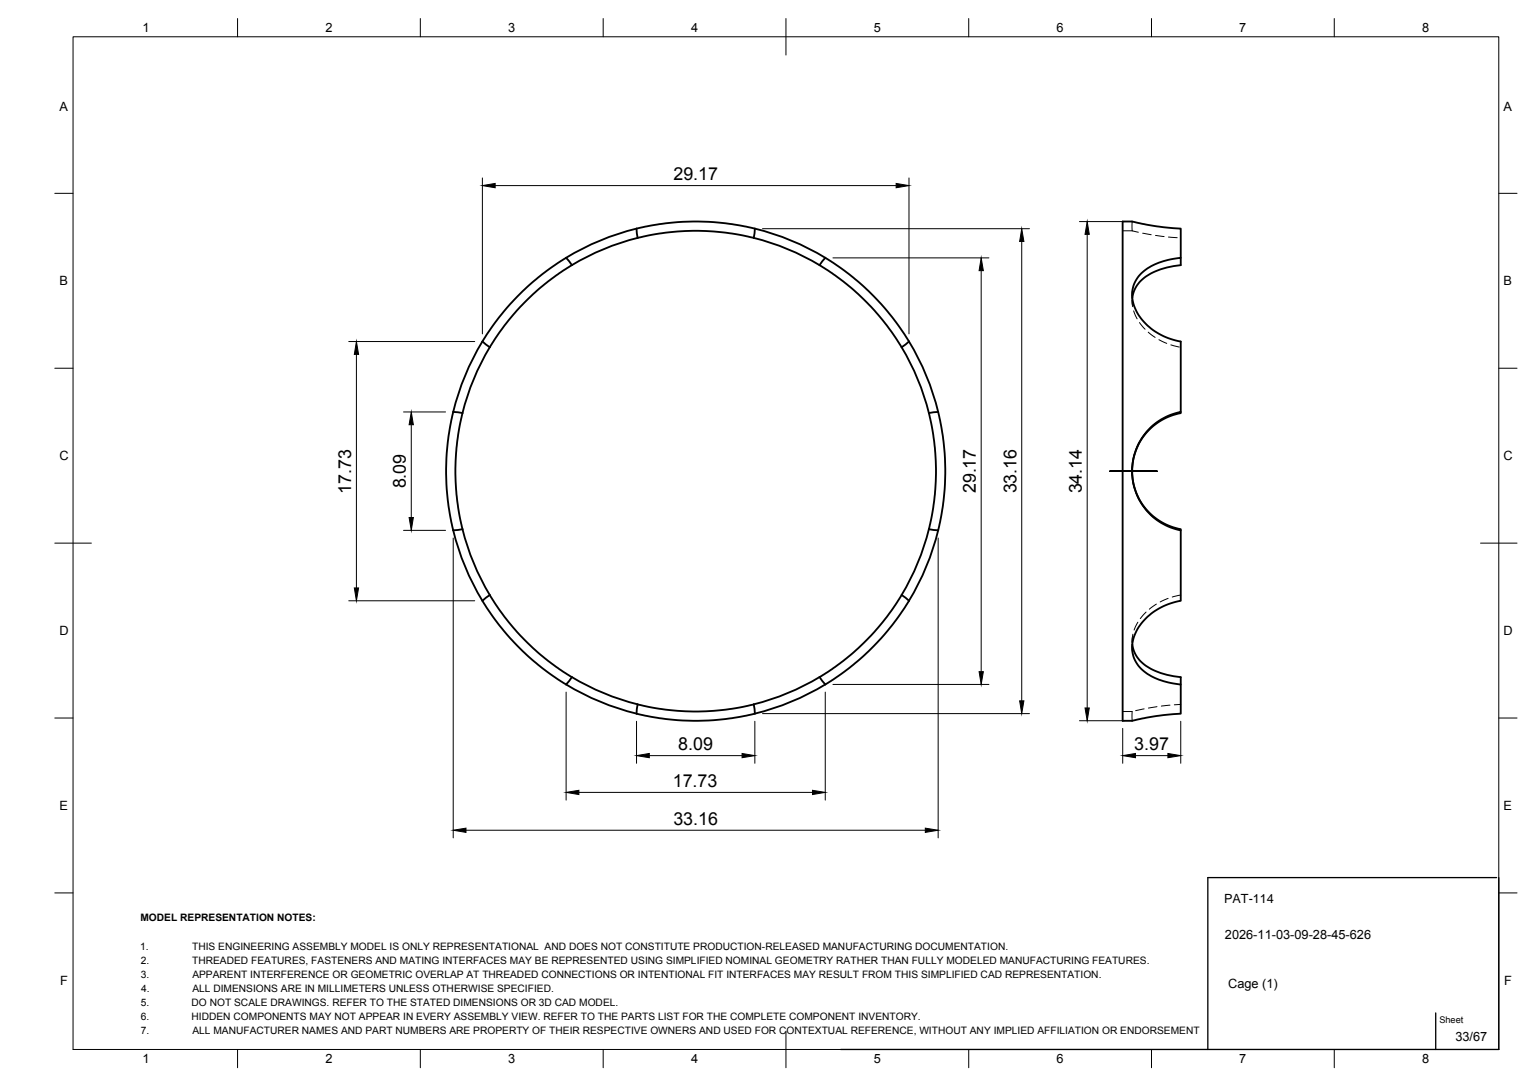
ISO-10303-21;
HEADER;
/* Generated by software containing ST-Developer
 * from STEP Tools, Inc. (www.steptools.com) 
 */

FILE_DESCRIPTION(
/* description */ ('Two-stage gear reducer in split housing'),
/* implementation_level */ '2;1');

FILE_NAME(
/* name */ 'Cage (1).step',
/* time_stamp */ '2026-10-28T03:22:31-07:00',
/* author */ (''),
/* organization */ (''),
/* preprocessor_version */ 'ST-DEVELOPER v20.2',
/* originating_system */ 'Autodesk Translation Framework v15.17.0.0',
/* authorisation */ '');

FILE_SCHEMA (('AUTOMOTIVE_DESIGN { 1 0 10303 214 3 1 1 }'));
ENDSEC;

DATA;
#10=MECHANICAL_DESIGN_GEOMETRIC_PRESENTATION_REPRESENTATION('',(#1273),#73366);
#945=B_SPLINE_CURVE_WITH_KNOTS('',3,(#24814,#24815,#24816,#24817,#24818,
#24819,#24820,#24821,#24822,#24823,#24824,#24825,#24826,#24827,#24828,#24829,
#24830,#24831,#24832,#24833,#24834,#24835),.UNSPECIFIED.,.F.,.F.,(4,2,2,
2,2,2,2,2,2,2,4),(0.0789094028588958,0.210573405340968,0.315860108011452,
0.421146810681936,0.522142632548711,0.623138454415485,0.72413427628226,
0.825130098149035,0.930416800819519,1.03570350349,1.16736750597208),
 .UNSPECIFIED.);
#946=B_SPLINE_CURVE_WITH_KNOTS('',3,(#24839,#24840,#24841,#24842,#24843,
#24844,#24845,#24846,#24847,#24848,#24849,#24850,#24851,#24852,#24853,#24854,
#24855,#24856,#24857,#24858,#24859,#24860),.UNSPECIFIED.,.F.,.F.,(4,2,2,
2,2,2,2,2,2,2,4),(0.0774793363974613,0.142088896491891,0.284177792983782,
0.411119756996526,0.514392970548519,0.617666184100513,0.720939397652506,
0.8242126112045,0.951154575217244,1.09324347170913,1.15785303180356),
 .UNSPECIFIED.);
#947=B_SPLINE_CURVE_WITH_KNOTS('',3,(#24866,#24867,#24868,#24869,#24870,
#24871,#24872,#24873,#24874,#24875,#24876,#24877,#24878,#24879,#24880,#24881,
#24882,#24883,#24884,#24885,#24886,#24887),.UNSPECIFIED.,.F.,.F.,(4,2,2,
2,2,2,2,2,2,2,4),(0.0774793363974613,0.142088896491891,0.284177792983782,
0.411119756996525,0.514392970548519,0.617666184100513,0.720939397652506,
0.8242126112045,0.951154575217243,1.09324347170913,1.15785303180356),
 .UNSPECIFIED.);
#948=B_SPLINE_CURVE_WITH_KNOTS('',3,(#24891,#24892,#24893,#24894,#24895,
#24896,#24897,#24898,#24899,#24900,#24901,#24902,#24903,#24904,#24905,#24906,
#24907,#24908,#24909,#24910,#24911,#24912),.UNSPECIFIED.,.F.,.F.,(4,2,2,
2,2,2,2,2,2,2,4),(0.0774793363974614,0.142088896491891,0.284177792983781,
0.411119756996525,0.514392970548519,0.617666184100512,0.720939397652506,
0.824212611204499,0.951154575217243,1.09324347170913,1.15785303180356),
 .UNSPECIFIED.);
#949=B_SPLINE_CURVE_WITH_KNOTS('',3,(#24916,#24917,#24918,#24919,#24920,
#24921,#24922,#24923,#24924,#24925,#24926,#24927),.UNSPECIFIED.,.F.,.F.,
(4,2,2,2,2,4),(0.0774793363974613,0.142088896491891,0.284177792983781,0.411119756996525,
0.514392970548519,0.617666184100512),.UNSPECIFIED.);
#950=B_SPLINE_CURVE_WITH_KNOTS('',3,(#24932,#24933,#24934,#24935,#24936,
#24937,#24938,#24939,#24940,#24941,#24942,#24943),.UNSPECIFIED.,.F.,.F.,
(4,2,2,2,2,4),(0.617666184100512,0.720939397652506,0.824212611204499,0.951154575217243,
1.09324347170913,1.15785303180356),.UNSPECIFIED.);
#951=B_SPLINE_CURVE_WITH_KNOTS('',3,(#24947,#24948,#24949,#24950,#24951,
#24952,#24953,#24954,#24955,#24956,#24957,#24958,#24959,#24960,#24961,#24962,
#24963,#24964,#24965,#24966,#24967,#24968),.UNSPECIFIED.,.F.,.F.,(4,2,2,
2,2,2,2,2,2,2,4),(0.0774793363974613,0.142088896491891,0.284177792983782,
0.411119756996526,0.514392970548519,0.617666184100513,0.720939397652507,
0.8242126112045,0.951154575217245,1.09324347170914,1.15785303180356),
 .UNSPECIFIED.);
#952=B_SPLINE_CURVE_WITH_KNOTS('',3,(#24972,#24973,#24974,#24975,#24976,
#24977,#24978,#24979,#24980,#24981,#24982,#24983,#24984,#24985,#24986,#24987,
#24988,#24989,#24990,#24991,#24992,#24993),.UNSPECIFIED.,.F.,.F.,(4,2,2,
2,2,2,2,2,2,2,4),(0.0774793363974613,0.142088896491891,0.284177792983782,
0.411119756996526,0.514392970548519,0.617666184100513,0.720939397652506,
0.824212611204499,0.951154575217243,1.09324347170913,1.15785303180356),
 .UNSPECIFIED.);
#953=B_SPLINE_CURVE_WITH_KNOTS('',3,(#24997,#24998,#24999,#25000,#25001,
#25002,#25003,#25004,#25005,#25006,#25007,#25008,#25009,#25010,#25011,#25012,
#25013,#25014,#25015,#25016,#25017,#25018),.UNSPECIFIED.,.F.,.F.,(4,2,2,
2,2,2,2,2,2,2,4),(0.0774793363974613,0.142088896491891,0.284177792983782,
0.411119756996526,0.514392970548519,0.617666184100513,0.720939397652506,
0.8242126112045,0.951154575217244,1.09324347170913,1.15785303180356),
 .UNSPECIFIED.);
#954=B_SPLINE_CURVE_WITH_KNOTS('',3,(#25022,#25023,#25024,#25025,#25026,
#25027,#25028,#25029,#25030,#25031,#25032,#25033,#25034,#25035,#25036,#25037,
#25038,#25039,#25040,#25041,#25042,#25043),.UNSPECIFIED.,.F.,.F.,(4,2,2,
2,2,2,2,2,2,2,4),(0.0774793363974613,0.142088896491891,0.284177792983782,
0.411119756996526,0.514392970548519,0.617666184100513,0.720939397652506,
0.8242126112045,0.951154575217243,1.09324347170913,1.15785303180356),
 .UNSPECIFIED.);
#955=B_SPLINE_CURVE_WITH_KNOTS('',3,(#25051,#25052,#25053,#25054,#25055,
#25056,#25057,#25058,#25059,#25060,#25061,#25062,#25063,#25064,#25065,#25066,
#25067,#25068,#25069,#25070,#25071,#25072),.UNSPECIFIED.,.F.,.F.,(4,2,2,
2,2,2,2,2,2,2,4),(0.0789094028588958,0.210573405340968,0.315860108011452,
0.421146810681936,0.522142632548711,0.623138454415485,0.72413427628226,
0.825130098149035,0.930416800819519,1.03570350349,1.16736750597208),
 .UNSPECIFIED.);
#956=B_SPLINE_CURVE_WITH_KNOTS('',3,(#25080,#25081,#25082,#25083,#25084,
#25085,#25086,#25087,#25088,#25089,#25090,#25091,#25092,#25093,#25094,#25095,
#25096,#25097,#25098,#25099,#25100,#25101),.UNSPECIFIED.,.F.,.F.,(4,2,2,
2,2,2,2,2,2,2,4),(0.0789094028588958,0.210573405340969,0.315860108011453,
0.421146810681937,0.522142632548712,0.623138454415486,0.724134276282261,
0.825130098149035,0.930416800819519,1.03570350349,1.16736750597208),
 .UNSPECIFIED.);
#957=B_SPLINE_CURVE_WITH_KNOTS('',3,(#25110,#25111,#25112,#25113,#25114,
#25115,#25116,#25117,#25118,#25119,#25120,#25121),.UNSPECIFIED.,.F.,.F.,
(4,2,2,2,2,4),(0.0789094028588958,0.210573405340968,0.315860108011452,0.421146810681937,
0.522142632548711,0.623138454415486),.UNSPECIFIED.);
#958=B_SPLINE_CURVE_WITH_KNOTS('',3,(#25123,#25124,#25125,#25126,#25127,
#25128,#25129,#25130,#25131,#25132,#25133,#25134),.UNSPECIFIED.,.F.,.F.,
(4,2,2,2,2,4),(0.623138454415486,0.72413427628226,0.825130098149035,0.930416800819519,
1.03570350349,1.16736750597208),.UNSPECIFIED.);
#959=B_SPLINE_CURVE_WITH_KNOTS('',3,(#25141,#25142,#25143,#25144,#25145,
#25146,#25147,#25148,#25149,#25150,#25151,#25152,#25153,#25154,#25155,#25156,
#25157,#25158,#25159,#25160,#25161,#25162),.UNSPECIFIED.,.F.,.F.,(4,2,2,
2,2,2,2,2,2,2,4),(0.0789094028588958,0.210573405340968,0.315860108011452,
0.421146810681936,0.522142632548711,0.623138454415486,0.72413427628226,
0.825130098149035,0.930416800819519,1.03570350349,1.16736750597208),
 .UNSPECIFIED.);
#960=B_SPLINE_CURVE_WITH_KNOTS('',3,(#25170,#25171,#25172,#25173,#25174,
#25175,#25176,#25177,#25178,#25179,#25180,#25181,#25182,#25183,#25184,#25185,
#25186,#25187,#25188,#25189,#25190,#25191),.UNSPECIFIED.,.F.,.F.,(4,2,2,
2,2,2,2,2,2,2,4),(0.0789094028588957,0.210573405340968,0.315860108011452,
0.421146810681936,0.522142632548711,0.623138454415485,0.72413427628226,
0.825130098149035,0.930416800819519,1.03570350349,1.16736750597207),
 .UNSPECIFIED.);
#961=B_SPLINE_CURVE_WITH_KNOTS('',3,(#25199,#25200,#25201,#25202,#25203,
#25204,#25205,#25206,#25207,#25208,#25209,#25210,#25211,#25212,#25213,#25214,
#25215,#25216,#25217,#25218,#25219,#25220),.UNSPECIFIED.,.F.,.F.,(4,2,2,
2,2,2,2,2,2,2,4),(0.0789094028588958,0.210573405340968,0.315860108011452,
0.421146810681936,0.522142632548711,0.623138454415486,0.72413427628226,
0.825130098149035,0.930416800819519,1.03570350349,1.16736750597208),
 .UNSPECIFIED.);
#962=B_SPLINE_CURVE_WITH_KNOTS('',3,(#25229,#25230,#25231,#25232,#25233,
#25234,#25235,#25236,#25237,#25238,#25239,#25240,#25241,#25242,#25243,#25244,
#25245,#25246,#25247,#25248,#25249,#25250),.UNSPECIFIED.,.F.,.F.,(4,2,2,
2,2,2,2,2,2,2,4),(0.0789094028588958,0.210573405340968,0.315860108011452,
0.421146810681936,0.522142632548711,0.623138454415485,0.72413427628226,
0.825130098149035,0.930416800819519,1.03570350349,1.16736750597208),
 .UNSPECIFIED.);
#1089=SPHERICAL_SURFACE('',#17603,0.412776);
#1090=SPHERICAL_SURFACE('',#17619,0.412776);
#1091=SPHERICAL_SURFACE('',#17624,0.412776);
#1092=SPHERICAL_SURFACE('',#17629,0.412776);
#1093=SPHERICAL_SURFACE('',#17634,0.412776);
#1094=SPHERICAL_SURFACE('',#17639,0.412776);
#1095=SPHERICAL_SURFACE('',#17644,0.412776);
#1096=SPHERICAL_SURFACE('',#17652,0.412776);
#1147=SHAPE_REPRESENTATION_RELATIONSHIP('SRR','None',#73636,#1203);
#1203=ADVANCED_BREP_SHAPE_REPRESENTATION('',(#1343),#73332);
#1273=STYLED_ITEM('',(#73988),#1343);
#1343=MANIFOLD_SOLID_BREP('Continuous crown cage',#16162);
#1532=FACE_BOUND('',#3461,.T.);
#1775=PLANE('',#17616);
#1776=PLANE('',#17621);
#1777=PLANE('',#17626);
#1778=PLANE('',#17631);
#1779=PLANE('',#17636);
#1780=PLANE('',#17641);
#1781=PLANE('',#17650);
#1782=PLANE('',#17654);
#1783=PLANE('',#17655);
#2372=FACE_OUTER_BOUND('',#3443,.T.);
#2373=FACE_OUTER_BOUND('',#3444,.T.);
#2374=FACE_OUTER_BOUND('',#3445,.T.);
#2375=FACE_OUTER_BOUND('',#3446,.T.);
#2376=FACE_OUTER_BOUND('',#3447,.T.);
#2377=FACE_OUTER_BOUND('',#3448,.T.);
#2378=FACE_OUTER_BOUND('',#3449,.T.);
#2379=FACE_OUTER_BOUND('',#3450,.T.);
#2380=FACE_OUTER_BOUND('',#3451,.T.);
#2381=FACE_OUTER_BOUND('',#3452,.T.);
#2382=FACE_OUTER_BOUND('',#3453,.T.);
#2383=FACE_OUTER_BOUND('',#3454,.T.);
#2384=FACE_OUTER_BOUND('',#3455,.T.);
#2385=FACE_OUTER_BOUND('',#3456,.T.);
#2386=FACE_OUTER_BOUND('',#3457,.T.);
#2387=FACE_OUTER_BOUND('',#3458,.T.);
#2388=FACE_OUTER_BOUND('',#3459,.T.);
#2389=FACE_OUTER_BOUND('',#3460,.T.);
#2390=FACE_OUTER_BOUND('',#3462,.T.);
#3443=EDGE_LOOP('',(#12093,#12094,#12095,#12096));
#3444=EDGE_LOOP('',(#12097,#12098,#12099,#12100,#12101,#12102,#12103,#12104,
#12105,#12106,#12107,#12108,#12109,#12110,#12111,#12112,#12113,#12114,#12115,
#12116));
#3445=EDGE_LOOP('',(#12117,#12118,#12119,#12120));
#3446=EDGE_LOOP('',(#12121,#12122,#12123,#12124));
#3447=EDGE_LOOP('',(#12125,#12126,#12127,#12128));
#3448=EDGE_LOOP('',(#12129,#12130,#12131,#12132));
#3449=EDGE_LOOP('',(#12133,#12134,#12135,#12136));
#3450=EDGE_LOOP('',(#12137,#12138,#12139,#12140,#12141,#12142));
#3451=EDGE_LOOP('',(#12143,#12144,#12145,#12146));
#3452=EDGE_LOOP('',(#12147,#12148,#12149,#12150));
#3453=EDGE_LOOP('',(#12151,#12152,#12153,#12154));
#3454=EDGE_LOOP('',(#12155,#12156,#12157,#12158));
#3455=EDGE_LOOP('',(#12159,#12160,#12161,#12162));
#3456=EDGE_LOOP('',(#12163,#12164,#12165,#12166));
#3457=EDGE_LOOP('',(#12167,#12168,#12169,#12170,#12171,#12172,#12173,#12174,
#12175,#12176,#12177,#12178,#12179,#12180,#12181,#12182,#12183,#12184,#12185,
#12186));
#3458=EDGE_LOOP('',(#12187,#12188,#12189,#12190));
#3459=EDGE_LOOP('',(#12191,#12192,#12193,#12194));
#3460=EDGE_LOOP('',(#12195));
#3461=EDGE_LOOP('',(#12196));
#3462=EDGE_LOOP('',(#12197,#12198,#12199,#12200));
#4449=LINE('',#24929,#5473);
#4450=LINE('',#25225,#5474);
#5473=VECTOR('',#20447,1.706752);
#5474=VECTOR('',#20524,1.643248);
#6490=CIRCLE('',#17604,0.405071403305639);
#6491=CIRCLE('',#17605,0.405071403305639);
#6492=CIRCLE('',#17607,1.706752);
#6493=CIRCLE('',#17608,1.706752);
#6494=CIRCLE('',#17609,1.706752);
#6495=CIRCLE('',#17610,1.706752);
#6496=CIRCLE('',#17611,1.706752);
#6497=CIRCLE('',#17612,1.706752);
#6498=CIRCLE('',#17613,1.706752);
#6499=CIRCLE('',#17614,1.706752);
#6500=CIRCLE('',#17615,1.706752);
#6501=CIRCLE('',#17617,1.643248);
#6502=CIRCLE('',#17618,0.405071403305639);
#6503=CIRCLE('',#17620,0.405071403305639);
#6504=CIRCLE('',#17622,1.643248);
#6505=CIRCLE('',#17623,0.405071403305639);
#6506=CIRCLE('',#17625,0.405071403305639);
#6507=CIRCLE('',#17627,1.643248);
#6508=CIRCLE('',#17628,0.405071403305639);
#6509=CIRCLE('',#17630,0.405071403305639);
#6510=CIRCLE('',#17632,1.643248);
#6511=CIRCLE('',#17633,0.405071403305639);
#6512=CIRCLE('',#17635,0.405071403305639);
#6513=CIRCLE('',#17637,1.643248);
#6514=CIRCLE('',#17638,0.405071403305639);
#6515=CIRCLE('',#17640,0.405071403305639);
#6516=CIRCLE('',#17642,1.643248);
#6517=CIRCLE('',#17643,0.405071403305639);
#6518=CIRCLE('',#17645,0.405071403305639);
#6519=CIRCLE('',#17647,1.643248);
#6520=CIRCLE('',#17648,1.643248);
#6521=CIRCLE('',#17649,1.643248);
#6522=CIRCLE('',#17651,0.405071403305639);
#6523=CIRCLE('',#17653,0.405071403305639);
#7369=VERTEX_POINT('',#24812);
#7370=VERTEX_POINT('',#24813);
#7371=VERTEX_POINT('',#24836);
#7372=VERTEX_POINT('',#24838);
#7373=VERTEX_POINT('',#24863);
#7374=VERTEX_POINT('',#24865);
#7375=VERTEX_POINT('',#24888);
#7376=VERTEX_POINT('',#24890);
#7377=VERTEX_POINT('',#24913);
#7378=VERTEX_POINT('',#24915);
#7379=VERTEX_POINT('',#24928);
#7380=VERTEX_POINT('',#24931);
#7381=VERTEX_POINT('',#24944);
#7382=VERTEX_POINT('',#24946);
#7383=VERTEX_POINT('',#24969);
#7384=VERTEX_POINT('',#24971);
#7385=VERTEX_POINT('',#24994);
#7386=VERTEX_POINT('',#24996);
#7387=VERTEX_POINT('',#25019);
#7388=VERTEX_POINT('',#25021);
#7389=VERTEX_POINT('',#25046);
#7390=VERTEX_POINT('',#25050);
#7391=VERTEX_POINT('',#25075);
#7392=VERTEX_POINT('',#25079);
#7393=VERTEX_POINT('',#25104);
#7394=VERTEX_POINT('',#25108);
#7395=VERTEX_POINT('',#25109);
#7396=VERTEX_POINT('',#25136);
#7397=VERTEX_POINT('',#25140);
#7398=VERTEX_POINT('',#25165);
#7399=VERTEX_POINT('',#25169);
#7400=VERTEX_POINT('',#25194);
#7401=VERTEX_POINT('',#25198);
#7402=VERTEX_POINT('',#25223);
#7403=VERTEX_POINT('',#25226);
#7404=VERTEX_POINT('',#25228);
#9100=EDGE_CURVE('',#7369,#7370,#945,.T.);
#9101=EDGE_CURVE('',#7371,#7369,#6490,.T.);
#9102=EDGE_CURVE('',#7372,#7371,#946,.T.);
#9103=EDGE_CURVE('',#7370,#7372,#6491,.T.);
#9104=EDGE_CURVE('',#7373,#7371,#6492,.T.);
#9105=EDGE_CURVE('',#7373,#7374,#947,.T.);
#9106=EDGE_CURVE('',#7375,#7374,#6493,.T.);
#9107=EDGE_CURVE('',#7375,#7376,#948,.T.);
#9108=EDGE_CURVE('',#7377,#7376,#6494,.T.);
#9109=EDGE_CURVE('',#7377,#7378,#949,.T.);
#9110=EDGE_CURVE('',#7378,#7379,#4449,.T.);
#9111=EDGE_CURVE('',#7379,#7379,#6495,.T.);
#9112=EDGE_CURVE('',#7378,#7380,#950,.T.);
#9113=EDGE_CURVE('',#7381,#7380,#6496,.T.);
#9114=EDGE_CURVE('',#7381,#7382,#951,.T.);
#9115=EDGE_CURVE('',#7383,#7382,#6497,.T.);
#9116=EDGE_CURVE('',#7383,#7384,#952,.T.);
#9117=EDGE_CURVE('',#7385,#7384,#6498,.T.);
#9118=EDGE_CURVE('',#7385,#7386,#953,.T.);
#9119=EDGE_CURVE('',#7387,#7386,#6499,.T.);
#9120=EDGE_CURVE('',#7387,#7388,#954,.T.);
#9121=EDGE_CURVE('',#7372,#7388,#6500,.T.);
#9122=EDGE_CURVE('',#7369,#7389,#6501,.T.);
#9123=EDGE_CURVE('',#7389,#7373,#6502,.T.);
#9124=EDGE_CURVE('',#7390,#7389,#955,.T.);
#9125=EDGE_CURVE('',#7374,#7390,#6503,.T.);
#9126=EDGE_CURVE('',#7390,#7391,#6504,.T.);
#9127=EDGE_CURVE('',#7391,#7375,#6505,.T.);
#9128=EDGE_CURVE('',#7392,#7391,#956,.T.);
#9129=EDGE_CURVE('',#7376,#7392,#6506,.T.);
#9130=EDGE_CURVE('',#7392,#7393,#6507,.T.);
#9131=EDGE_CURVE('',#7393,#7377,#6508,.T.);
#9132=EDGE_CURVE('',#7394,#7395,#957,.T.);
#9133=EDGE_CURVE('',#7380,#7394,#6509,.T.);
#9134=EDGE_CURVE('',#7395,#7393,#958,.T.);
#9135=EDGE_CURVE('',#7394,#7396,#6510,.T.);
#9136=EDGE_CURVE('',#7396,#7381,#6511,.T.);
#9137=EDGE_CURVE('',#7397,#7396,#959,.T.);
#9138=EDGE_CURVE('',#7382,#7397,#6512,.T.);
#9139=EDGE_CURVE('',#7397,#7398,#6513,.T.);
#9140=EDGE_CURVE('',#7398,#7383,#6514,.T.);
#9141=EDGE_CURVE('',#7399,#7398,#960,.T.);
#9142=EDGE_CURVE('',#7384,#7399,#6515,.T.);
#9143=EDGE_CURVE('',#7399,#7400,#6516,.T.);
#9144=EDGE_CURVE('',#7400,#7385,#6517,.T.);
#9145=EDGE_CURVE('',#7401,#7400,#961,.T.);
#9146=EDGE_CURVE('',#7386,#7401,#6518,.T.);
#9147=EDGE_CURVE('',#7402,#7402,#6519,.T.);
#9148=EDGE_CURVE('',#7402,#7395,#4450,.T.);
#9149=EDGE_CURVE('',#7403,#7370,#6520,.T.);
#9150=EDGE_CURVE('',#7403,#7404,#962,.T.);
#9151=EDGE_CURVE('',#7401,#7404,#6521,.T.);
#9152=EDGE_CURVE('',#7388,#7403,#6522,.T.);
#9153=EDGE_CURVE('',#7404,#7387,#6523,.T.);
#12093=ORIENTED_EDGE('',*,*,#9100,.F.);
#12094=ORIENTED_EDGE('',*,*,#9101,.F.);
#12095=ORIENTED_EDGE('',*,*,#9102,.F.);
#12096=ORIENTED_EDGE('',*,*,#9103,.F.);
#12097=ORIENTED_EDGE('',*,*,#9102,.T.);
#12098=ORIENTED_EDGE('',*,*,#9104,.F.);
#12099=ORIENTED_EDGE('',*,*,#9105,.T.);
#12100=ORIENTED_EDGE('',*,*,#9106,.F.);
#12101=ORIENTED_EDGE('',*,*,#9107,.T.);
#12102=ORIENTED_EDGE('',*,*,#9108,.F.);
#12103=ORIENTED_EDGE('',*,*,#9109,.T.);
#12104=ORIENTED_EDGE('',*,*,#9110,.T.);
#12105=ORIENTED_EDGE('',*,*,#9111,.F.);
#12106=ORIENTED_EDGE('',*,*,#9110,.F.);
#12107=ORIENTED_EDGE('',*,*,#9112,.T.);
#12108=ORIENTED_EDGE('',*,*,#9113,.F.);
#12109=ORIENTED_EDGE('',*,*,#9114,.T.);
#12110=ORIENTED_EDGE('',*,*,#9115,.F.);
#12111=ORIENTED_EDGE('',*,*,#9116,.T.);
#12112=ORIENTED_EDGE('',*,*,#9117,.F.);
#12113=ORIENTED_EDGE('',*,*,#9118,.T.);
#12114=ORIENTED_EDGE('',*,*,#9119,.F.);
#12115=ORIENTED_EDGE('',*,*,#9120,.T.);
#12116=ORIENTED_EDGE('',*,*,#9121,.F.);
#12117=ORIENTED_EDGE('',*,*,#9101,.T.);
#12118=ORIENTED_EDGE('',*,*,#9122,.T.);
#12119=ORIENTED_EDGE('',*,*,#9123,.T.);
#12120=ORIENTED_EDGE('',*,*,#9104,.T.);
#12121=ORIENTED_EDGE('',*,*,#9124,.F.);
#12122=ORIENTED_EDGE('',*,*,#9125,.F.);
#12123=ORIENTED_EDGE('',*,*,#9105,.F.);
#12124=ORIENTED_EDGE('',*,*,#9123,.F.);
#12125=ORIENTED_EDGE('',*,*,#9125,.T.);
#12126=ORIENTED_EDGE('',*,*,#9126,.T.);
#12127=ORIENTED_EDGE('',*,*,#9127,.T.);
#12128=ORIENTED_EDGE('',*,*,#9106,.T.);
#12129=ORIENTED_EDGE('',*,*,#9128,.F.);
#12130=ORIENTED_EDGE('',*,*,#9129,.F.);
#12131=ORIENTED_EDGE('',*,*,#9107,.F.);
#12132=ORIENTED_EDGE('',*,*,#9127,.F.);
#12133=ORIENTED_EDGE('',*,*,#9129,.T.);
#12134=ORIENTED_EDGE('',*,*,#9130,.T.);
#12135=ORIENTED_EDGE('',*,*,#9131,.T.);
#12136=ORIENTED_EDGE('',*,*,#9108,.T.);
#12137=ORIENTED_EDGE('',*,*,#9132,.F.);
#12138=ORIENTED_EDGE('',*,*,#9133,.F.);
#12139=ORIENTED_EDGE('',*,*,#9112,.F.);
#12140=ORIENTED_EDGE('',*,*,#9109,.F.);
#12141=ORIENTED_EDGE('',*,*,#9131,.F.);
#12142=ORIENTED_EDGE('',*,*,#9134,.F.);
#12143=ORIENTED_EDGE('',*,*,#9133,.T.);
#12144=ORIENTED_EDGE('',*,*,#9135,.T.);
#12145=ORIENTED_EDGE('',*,*,#9136,.T.);
#12146=ORIENTED_EDGE('',*,*,#9113,.T.);
#12147=ORIENTED_EDGE('',*,*,#9137,.F.);
#12148=ORIENTED_EDGE('',*,*,#9138,.F.);
#12149=ORIENTED_EDGE('',*,*,#9114,.F.);
#12150=ORIENTED_EDGE('',*,*,#9136,.F.);
#12151=ORIENTED_EDGE('',*,*,#9138,.T.);
#12152=ORIENTED_EDGE('',*,*,#9139,.T.);
#12153=ORIENTED_EDGE('',*,*,#9140,.T.);
#12154=ORIENTED_EDGE('',*,*,#9115,.T.);
#12155=ORIENTED_EDGE('',*,*,#9141,.F.);
#12156=ORIENTED_EDGE('',*,*,#9142,.F.);
#12157=ORIENTED_EDGE('',*,*,#9116,.F.);
#12158=ORIENTED_EDGE('',*,*,#9140,.F.);
#12159=ORIENTED_EDGE('',*,*,#9142,.T.);
#12160=ORIENTED_EDGE('',*,*,#9143,.T.);
#12161=ORIENTED_EDGE('',*,*,#9144,.T.);
#12162=ORIENTED_EDGE('',*,*,#9117,.T.);
#12163=ORIENTED_EDGE('',*,*,#9118,.F.);
#12164=ORIENTED_EDGE('',*,*,#9144,.F.);
#12165=ORIENTED_EDGE('',*,*,#9145,.F.);
#12166=ORIENTED_EDGE('',*,*,#9146,.F.);
#12167=ORIENTED_EDGE('',*,*,#9147,.F.);
#12168=ORIENTED_EDGE('',*,*,#9148,.T.);
#12169=ORIENTED_EDGE('',*,*,#9134,.T.);
#12170=ORIENTED_EDGE('',*,*,#9130,.F.);
#12171=ORIENTED_EDGE('',*,*,#9128,.T.);
#12172=ORIENTED_EDGE('',*,*,#9126,.F.);
#12173=ORIENTED_EDGE('',*,*,#9124,.T.);
#12174=ORIENTED_EDGE('',*,*,#9122,.F.);
#12175=ORIENTED_EDGE('',*,*,#9100,.T.);
#12176=ORIENTED_EDGE('',*,*,#9149,.F.);
#12177=ORIENTED_EDGE('',*,*,#9150,.T.);
#12178=ORIENTED_EDGE('',*,*,#9151,.F.);
#12179=ORIENTED_EDGE('',*,*,#9145,.T.);
#12180=ORIENTED_EDGE('',*,*,#9143,.F.);
#12181=ORIENTED_EDGE('',*,*,#9141,.T.);
#12182=ORIENTED_EDGE('',*,*,#9139,.F.);
#12183=ORIENTED_EDGE('',*,*,#9137,.T.);
#12184=ORIENTED_EDGE('',*,*,#9135,.F.);
#12185=ORIENTED_EDGE('',*,*,#9132,.T.);
#12186=ORIENTED_EDGE('',*,*,#9148,.F.);
#12187=ORIENTED_EDGE('',*,*,#9103,.T.);
#12188=ORIENTED_EDGE('',*,*,#9121,.T.);
#12189=ORIENTED_EDGE('',*,*,#9152,.T.);
#12190=ORIENTED_EDGE('',*,*,#9149,.T.);
#12191=ORIENTED_EDGE('',*,*,#9120,.F.);
#12192=ORIENTED_EDGE('',*,*,#9153,.F.);
#12193=ORIENTED_EDGE('',*,*,#9150,.F.);
#12194=ORIENTED_EDGE('',*,*,#9152,.F.);
#12195=ORIENTED_EDGE('',*,*,#9111,.T.);
#12196=ORIENTED_EDGE('',*,*,#9147,.T.);
#12197=ORIENTED_EDGE('',*,*,#9146,.T.);
#12198=ORIENTED_EDGE('',*,*,#9151,.T.);
#12199=ORIENTED_EDGE('',*,*,#9153,.T.);
#12200=ORIENTED_EDGE('',*,*,#9119,.T.);
#15067=CYLINDRICAL_SURFACE('',#17606,1.706752);
#15068=CYLINDRICAL_SURFACE('',#17646,1.643248);
#15579=ADVANCED_FACE('',(#2372),#1089,.F.);
#15580=ADVANCED_FACE('',(#2373),#15067,.T.);
#15581=ADVANCED_FACE('',(#2374),#1775,.T.);
#15582=ADVANCED_FACE('',(#2375),#1090,.F.);
#15583=ADVANCED_FACE('',(#2376),#1776,.T.);
#15584=ADVANCED_FACE('',(#2377),#1091,.F.);
#15585=ADVANCED_FACE('',(#2378),#1777,.T.);
#15586=ADVANCED_FACE('',(#2379),#1092,.F.);
#15587=ADVANCED_FACE('',(#2380),#1778,.T.);
#15588=ADVANCED_FACE('',(#2381),#1093,.F.);
#15589=ADVANCED_FACE('',(#2382),#1779,.T.);
#15590=ADVANCED_FACE('',(#2383),#1094,.F.);
#15591=ADVANCED_FACE('',(#2384),#1780,.T.);
#15592=ADVANCED_FACE('',(#2385),#1095,.F.);
#15593=ADVANCED_FACE('',(#2386),#15068,.F.);
#15594=ADVANCED_FACE('',(#2387),#1781,.T.);
#15595=ADVANCED_FACE('',(#2388),#1096,.F.);
#15596=ADVANCED_FACE('',(#2389,#1532),#1782,.T.);
#15597=ADVANCED_FACE('',(#2390),#1783,.T.);
#16162=CLOSED_SHELL('',(#15579,#15580,#15581,#15582,#15583,#15584,#15585,
#15586,#15587,#15588,#15589,#15590,#15591,#15592,#15593,#15594,#15595,#15596,
#15597));
#17602=AXIS2_PLACEMENT_3D('',#24810,#20431,#20432);
#17603=AXIS2_PLACEMENT_3D('',#24811,#20433,#20434);
#17604=AXIS2_PLACEMENT_3D('',#24837,#20435,#20436);
#17605=AXIS2_PLACEMENT_3D('',#24861,#20437,#20438);
#17606=AXIS2_PLACEMENT_3D('',#24862,#20439,#20440);
#17607=AXIS2_PLACEMENT_3D('',#24864,#20441,#20442);
#17608=AXIS2_PLACEMENT_3D('',#24889,#20443,#20444);
#17609=AXIS2_PLACEMENT_3D('',#24914,#20445,#20446);
#17610=AXIS2_PLACEMENT_3D('',#24930,#20448,#20449);
#17611=AXIS2_PLACEMENT_3D('',#24945,#20450,#20451);
#17612=AXIS2_PLACEMENT_3D('',#24970,#20452,#20453);
#17613=AXIS2_PLACEMENT_3D('',#24995,#20454,#20455);
#17614=AXIS2_PLACEMENT_3D('',#25020,#20456,#20457);
#17615=AXIS2_PLACEMENT_3D('',#25044,#20458,#20459);
#17616=AXIS2_PLACEMENT_3D('',#25045,#20460,#20461);
#17617=AXIS2_PLACEMENT_3D('',#25047,#20462,#20463);
#17618=AXIS2_PLACEMENT_3D('',#25048,#20464,#20465);
#17619=AXIS2_PLACEMENT_3D('',#25049,#20466,#20467);
#17620=AXIS2_PLACEMENT_3D('',#25073,#20468,#20469);
#17621=AXIS2_PLACEMENT_3D('',#25074,#20470,#20471);
#17622=AXIS2_PLACEMENT_3D('',#25076,#20472,#20473);
#17623=AXIS2_PLACEMENT_3D('',#25077,#20474,#20475);
#17624=AXIS2_PLACEMENT_3D('',#25078,#20476,#20477);
#17625=AXIS2_PLACEMENT_3D('',#25102,#20478,#20479);
#17626=AXIS2_PLACEMENT_3D('',#25103,#20480,#20481);
#17627=AXIS2_PLACEMENT_3D('',#25105,#20482,#20483);
#17628=AXIS2_PLACEMENT_3D('',#25106,#20484,#20485);
#17629=AXIS2_PLACEMENT_3D('',#25107,#20486,#20487);
#17630=AXIS2_PLACEMENT_3D('',#25122,#20488,#20489);
#17631=AXIS2_PLACEMENT_3D('',#25135,#20490,#20491);
#17632=AXIS2_PLACEMENT_3D('',#25137,#20492,#20493);
#17633=AXIS2_PLACEMENT_3D('',#25138,#20494,#20495);
#17634=AXIS2_PLACEMENT_3D('',#25139,#20496,#20497);
#17635=AXIS2_PLACEMENT_3D('',#25163,#20498,#20499);
#17636=AXIS2_PLACEMENT_3D('',#25164,#20500,#20501);
#17637=AXIS2_PLACEMENT_3D('',#25166,#20502,#20503);
#17638=AXIS2_PLACEMENT_3D('',#25167,#20504,#20505);
#17639=AXIS2_PLACEMENT_3D('',#25168,#20506,#20507);
#17640=AXIS2_PLACEMENT_3D('',#25192,#20508,#20509);
#17641=AXIS2_PLACEMENT_3D('',#25193,#20510,#20511);
#17642=AXIS2_PLACEMENT_3D('',#25195,#20512,#20513);
#17643=AXIS2_PLACEMENT_3D('',#25196,#20514,#20515);
#17644=AXIS2_PLACEMENT_3D('',#25197,#20516,#20517);
#17645=AXIS2_PLACEMENT_3D('',#25221,#20518,#20519);
#17646=AXIS2_PLACEMENT_3D('',#25222,#20520,#20521);
#17647=AXIS2_PLACEMENT_3D('',#25224,#20522,#20523);
#17648=AXIS2_PLACEMENT_3D('',#25227,#20525,#20526);
#17649=AXIS2_PLACEMENT_3D('',#25251,#20527,#20528);
#17650=AXIS2_PLACEMENT_3D('',#25252,#20529,#20530);
#17651=AXIS2_PLACEMENT_3D('',#25253,#20531,#20532);
#17652=AXIS2_PLACEMENT_3D('',#25254,#20533,#20534);
#17653=AXIS2_PLACEMENT_3D('',#25255,#20535,#20536);
#17654=AXIS2_PLACEMENT_3D('',#25256,#20537,#20538);
#17655=AXIS2_PLACEMENT_3D('',#25257,#20539,#20540);
#20431=DIRECTION('axis',(0.,0.,1.));
#20432=DIRECTION('refdir',(1.,0.,0.));
#20433=DIRECTION('center_axis',(0.,0.,1.));
#20434=DIRECTION('ref_axis',(1.,0.,0.));
#20435=DIRECTION('center_axis',(0.,-1.,0.));
#20436=DIRECTION('ref_axis',(0.,0.,-1.));
#20437=DIRECTION('center_axis',(0.,-1.,0.));
#20438=DIRECTION('ref_axis',(0.,0.,-1.));
#20439=DIRECTION('center_axis',(0.,1.,0.));
#20440=DIRECTION('ref_axis',(1.,0.,0.));
#20441=DIRECTION('center_axis',(0.,1.,0.));
#20442=DIRECTION('ref_axis',(1.,0.,0.));
#20443=DIRECTION('center_axis',(0.,1.,0.));
#20444=DIRECTION('ref_axis',(1.,0.,0.));
#20445=DIRECTION('center_axis',(0.,1.,0.));
#20446=DIRECTION('ref_axis',(1.,0.,0.));
#20447=DIRECTION('',(0.,-1.,0.));
#20448=DIRECTION('center_axis',(0.,-1.,0.));
#20449=DIRECTION('ref_axis',(1.,0.,0.));
#20450=DIRECTION('center_axis',(0.,1.,0.));
#20451=DIRECTION('ref_axis',(1.,0.,0.));
#20452=DIRECTION('center_axis',(0.,1.,0.));
#20453=DIRECTION('ref_axis',(1.,0.,0.));
#20454=DIRECTION('center_axis',(0.,1.,0.));
#20455=DIRECTION('ref_axis',(1.,0.,0.));
#20456=DIRECTION('center_axis',(0.,1.,0.));
#20457=DIRECTION('ref_axis',(1.,0.,0.));
#20458=DIRECTION('center_axis',(0.,1.,0.));
#20459=DIRECTION('ref_axis',(1.,0.,0.));
#20460=DIRECTION('center_axis',(0.,1.,0.));
#20461=DIRECTION('ref_axis',(1.,0.,0.));
#20462=DIRECTION('center_axis',(0.,-1.,0.));
#20463=DIRECTION('ref_axis',(1.,0.,0.));
#20464=DIRECTION('center_axis',(0.,-1.,0.));
#20465=DIRECTION('ref_axis',(0.,0.,-1.));
#20466=DIRECTION('center_axis',(6.12323399573677E-17,0.,1.));
#20467=DIRECTION('ref_axis',(1.,0.,0.));
#20468=DIRECTION('center_axis',(0.,-1.,0.));
#20469=DIRECTION('ref_axis',(0.,0.,-1.));
#20470=DIRECTION('center_axis',(0.,1.,0.));
#20471=DIRECTION('ref_axis',(1.,0.,0.));
#20472=DIRECTION('center_axis',(0.,-1.,0.));
#20473=DIRECTION('ref_axis',(1.,0.,0.));
#20474=DIRECTION('center_axis',(0.,-1.,0.));
#20475=DIRECTION('ref_axis',(0.,0.,-1.));
#20476=DIRECTION('center_axis',(0.,0.,1.));
#20477=DIRECTION('ref_axis',(1.,0.,0.));
#20478=DIRECTION('center_axis',(0.,-1.,0.));
#20479=DIRECTION('ref_axis',(0.,0.,-1.));
#20480=DIRECTION('center_axis',(0.,1.,0.));
#20481=DIRECTION('ref_axis',(1.,0.,0.));
#20482=DIRECTION('center_axis',(0.,-1.,0.));
#20483=DIRECTION('ref_axis',(1.,0.,0.));
#20484=DIRECTION('center_axis',(0.,-1.,0.));
#20485=DIRECTION('ref_axis',(0.,0.,-1.));
#20486=DIRECTION('center_axis',(0.,0.,1.));
#20487=DIRECTION('ref_axis',(1.,0.,0.));
#20488=DIRECTION('center_axis',(0.,-1.,0.));
#20489=DIRECTION('ref_axis',(0.,0.,-1.));
#20490=DIRECTION('center_axis',(0.,1.,0.));
#20491=DIRECTION('ref_axis',(1.,0.,0.));
#20492=DIRECTION('center_axis',(0.,-1.,0.));
#20493=DIRECTION('ref_axis',(1.,0.,0.));
#20494=DIRECTION('center_axis',(0.,-1.,0.));
#20495=DIRECTION('ref_axis',(0.,0.,-1.));
#20496=DIRECTION('center_axis',(0.,0.,1.));
#20497=DIRECTION('ref_axis',(1.,0.,0.));
#20498=DIRECTION('center_axis',(0.,-1.,0.));
#20499=DIRECTION('ref_axis',(0.,0.,-1.));
#20500=DIRECTION('center_axis',(0.,1.,0.));
#20501=DIRECTION('ref_axis',(1.,0.,0.));
#20502=DIRECTION('center_axis',(0.,-1.,0.));
#20503=DIRECTION('ref_axis',(1.,0.,0.));
#20504=DIRECTION('center_axis',(0.,-1.,0.));
#20505=DIRECTION('ref_axis',(0.,0.,-1.));
#20506=DIRECTION('center_axis',(6.12323399573676E-17,0.,1.));
#20507=DIRECTION('ref_axis',(1.,0.,0.));
#20508=DIRECTION('center_axis',(0.,-1.,0.));
#20509=DIRECTION('ref_axis',(0.,0.,-1.));
#20510=DIRECTION('center_axis',(0.,1.,0.));
#20511=DIRECTION('ref_axis',(1.,0.,0.));
#20512=DIRECTION('center_axis',(0.,-1.,0.));
#20513=DIRECTION('ref_axis',(1.,0.,0.));
#20514=DIRECTION('center_axis',(0.,-1.,0.));
#20515=DIRECTION('ref_axis',(0.,0.,-1.));
#20516=DIRECTION('center_axis',(0.,0.,1.));
#20517=DIRECTION('ref_axis',(1.,0.,0.));
#20518=DIRECTION('center_axis',(0.,-1.,0.));
#20519=DIRECTION('ref_axis',(0.,0.,-1.));
#20520=DIRECTION('center_axis',(0.,1.,0.));
#20521=DIRECTION('ref_axis',(1.,0.,0.));
#20522=DIRECTION('center_axis',(0.,1.,0.));
#20523=DIRECTION('ref_axis',(1.,0.,0.));
#20524=DIRECTION('',(0.,1.,0.));
#20525=DIRECTION('center_axis',(0.,-1.,0.));
#20526=DIRECTION('ref_axis',(1.,0.,0.));
#20527=DIRECTION('center_axis',(0.,-1.,0.));
#20528=DIRECTION('ref_axis',(1.,0.,0.));
#20529=DIRECTION('center_axis',(0.,1.,0.));
#20530=DIRECTION('ref_axis',(1.,0.,0.));
#20531=DIRECTION('center_axis',(0.,-1.,0.));
#20532=DIRECTION('ref_axis',(0.,0.,-1.));
#20533=DIRECTION('center_axis',(0.,0.,1.));
#20534=DIRECTION('ref_axis',(1.,0.,0.));
#20535=DIRECTION('center_axis',(0.,-1.,0.));
#20536=DIRECTION('ref_axis',(0.,0.,-1.));
#20537=DIRECTION('center_axis',(0.,-1.,0.));
#20538=DIRECTION('ref_axis',(-1.,0.,0.));
#20539=DIRECTION('center_axis',(0.,1.,0.));
#20540=DIRECTION('ref_axis',(1.,0.,0.));
#24810=CARTESIAN_POINT('',(0.,0.,0.));
#24811=CARTESIAN_POINT('Origin',(1.18440385848747,0.,1.18440385848747));
#24812=CARTESIAN_POINT('',(0.846804978391753,-0.07938,1.40825612658882));
#24813=CARTESIAN_POINT('',(1.40825612658882,-0.07938,0.846804978391754));
#24814=CARTESIAN_POINT('Ctrl Pts',(0.846804978391752,-0.0793800000000001,
1.40825612658882));
#24815=CARTESIAN_POINT('Ctrl Pts',(0.854205272175554,-0.123401821157026,
1.40380622184538));
#24816=CARTESIAN_POINT('Ctrl Pts',(0.867957148219441,-0.166543350814306,
1.39550172959303));
#24817=CARTESIAN_POINT('Ctrl Pts',(0.902193646979982,-0.237231147975234,
1.3735491215176));
#24818=CARTESIAN_POINT('Ctrl Pts',(0.920778333482564,-0.266264900654909,
1.36127834356734));
#24819=CARTESIAN_POINT('Ctrl Pts',(0.962485392528369,-0.317195968905306,
1.33211611256184));
#24820=CARTESIAN_POINT('Ctrl Pts',(0.985600426557816,-0.33909093068465,
1.31521005565926));
#24821=CARTESIAN_POINT('Ctrl Pts',(1.03253285680459,-0.373586846396559,
1.27866649102984));
#24822=CARTESIAN_POINT('Ctrl Pts',(1.05871835910697,-0.388086240756494,
1.25722555095714));
#24823=CARTESIAN_POINT('Ctrl Pts',(1.11153475808518,-0.407068917407805,
1.2107812086231));
#24824=CARTESIAN_POINT('Ctrl Pts',(1.13814686046673,-0.411552957311693,
1.18575674747573));
#24825=CARTESIAN_POINT('Ctrl Pts',(1.18575674747573,-0.411552957311693,
1.13814686046673));
#24826=CARTESIAN_POINT('Ctrl Pts',(1.2107812086231,-0.407068917407805,1.11153475808518));
#24827=CARTESIAN_POINT('Ctrl Pts',(1.25722555095713,-0.388086240756494,
1.05871835910697));
#24828=CARTESIAN_POINT('Ctrl Pts',(1.27866649102984,-0.373586846396559,
1.03253285680459));
#24829=CARTESIAN_POINT('Ctrl Pts',(1.31521005565926,-0.33909093068465,0.985600426557816));
#24830=CARTESIAN_POINT('Ctrl Pts',(1.33211611256184,-0.317195968905306,
0.962485392528369));
#24831=CARTESIAN_POINT('Ctrl Pts',(1.36127834356734,-0.266264900654909,
0.920778333482565));
#24832=CARTESIAN_POINT('Ctrl Pts',(1.3735491215176,-0.237231147975234,0.902193646979983));
#24833=CARTESIAN_POINT('Ctrl Pts',(1.39550172959303,-0.166543350814306,
0.867957148219442));
#24834=CARTESIAN_POINT('Ctrl Pts',(1.40380622184538,-0.123401821157026,
0.854205272175555));
#24835=CARTESIAN_POINT('Ctrl Pts',(1.40825612658882,-0.0793800000000001,
0.846804978391753));
#24836=CARTESIAN_POINT('',(0.886256117232623,-0.07938,1.45861320581289));
#24837=CARTESIAN_POINT('Origin',(1.18440385848747,-0.07938,1.18440385848747));
#24838=CARTESIAN_POINT('',(1.45861320581289,-0.07938,0.886256117232624));
#24839=CARTESIAN_POINT('Ctrl Pts',(1.45861320581289,-0.0793800000000001,
0.886256117232623));
#24840=CARTESIAN_POINT('Ctrl Pts',(1.45630208793976,-0.101649918886749,
0.890059788636852));
#24841=CARTESIAN_POINT('Ctrl Pts',(1.45296717977858,-0.123823518623746,
0.895520212222107));
#24842=CARTESIAN_POINT('Ctrl Pts',(1.43904931717599,-0.192480977588836,
0.917859913453975));
#24843=CARTESIAN_POINT('Ctrl Pts',(1.4243271592157,-0.236152929235938,0.940896403863072));
#24844=CARTESIAN_POINT('Ctrl Pts',(1.39055359345152,-0.303141259068212,
0.990027513266106));
#24845=CARTESIAN_POINT('Ctrl Pts',(1.36743459453896,-0.335108247315849,
1.02199477007745));
#24846=CARTESIAN_POINT('Ctrl Pts',(1.32643091652006,-0.373243761060364,
1.07446535104584));
#24847=CARTESIAN_POINT('Ctrl Pts',(1.30441816675528,-0.387888272594439,
1.10126842659597));
#24848=CARTESIAN_POINT('Ctrl Pts',(1.25681160160691,-0.407041111792943,
1.15530234155453));
#24849=CARTESIAN_POINT('Ctrl Pts',(1.23119764287622,-0.411552957311693,
1.18251418313119));
#24850=CARTESIAN_POINT('Ctrl Pts',(1.18251418313119,-0.411552957311693,
1.23119764287622));
#24851=CARTESIAN_POINT('Ctrl Pts',(1.15530234155453,-0.407041111792943,
1.25681160160691));
#24852=CARTESIAN_POINT('Ctrl Pts',(1.10126842659597,-0.387888272594439,
1.30441816675528));
#24853=CARTESIAN_POINT('Ctrl Pts',(1.07446535104584,-0.373243761060364,
1.32643091652006));
#24854=CARTESIAN_POINT('Ctrl Pts',(1.02199477007745,-0.335108247315848,
1.36743459453896));
#24855=CARTESIAN_POINT('Ctrl Pts',(0.990027513266105,-0.303141259068211,
1.39055359345152));
#24856=CARTESIAN_POINT('Ctrl Pts',(0.940896403863071,-0.236152929235937,
1.42432715921571));
#24857=CARTESIAN_POINT('Ctrl Pts',(0.917859913453974,-0.192480977588835,
1.43904931717599));
#24858=CARTESIAN_POINT('Ctrl Pts',(0.895520212222106,-0.123823518623745,
1.45296717977858));
#24859=CARTESIAN_POINT('Ctrl Pts',(0.890059788636851,-0.101649918886749,
1.45630208793976));
#24860=CARTESIAN_POINT('Ctrl Pts',(0.886256117232622,-0.0793800000000001,
1.45861320581289));
#24861=CARTESIAN_POINT('Origin',(1.18440385848747,-0.07938,1.18440385848747));
#24862=CARTESIAN_POINT('Origin',(0.,-0.27783,0.));
#24863=CARTESIAN_POINT('',(0.404717578595295,-0.07938,1.65807299932179));
#24864=CARTESIAN_POINT('Origin',(0.,-0.07938,0.));
#24865=CARTESIAN_POINT('',(-0.404717578595296,-0.07938,1.65807299932179));
#24866=CARTESIAN_POINT('Ctrl Pts',(0.404717578595296,-0.0793800000000001,
1.65807299932179));
#24867=CARTESIAN_POINT('Ctrl Pts',(0.400393769631747,-0.101649918886749,
1.65912839404491));
#24868=CARTESIAN_POINT('Ctrl Pts',(0.394174530911058,-0.123823518623745,
1.66063136041479));
#24869=CARTESIAN_POINT('Ctrl Pts',(0.368536561654407,-0.192480977588835,
1.66658649961961));
#24870=CARTESIAN_POINT('Ctrl Pts',(0.341837165343982,-0.236152929235937,
1.67246562047521));
#24871=CARTESIAN_POINT('Ctrl Pts',(0.283214707341173,-0.303141259068211,
1.68332504372461));
#24872=CARTESIAN_POINT('Ctrl Pts',(0.244262842368623,-0.335108247315849,
1.68958170688653));
#24873=CARTESIAN_POINT('Ctrl Pts',(0.178166559972324,-0.373243761060364,
1.69769003172132));
#24874=CARTESIAN_POINT('Ctrl Pts',(0.143648558862931,-0.387888272594439,
1.70107730356824));
#24875=CARTESIAN_POINT('Ctrl Pts',(0.0717778861362652,-0.407041111792943,
1.70562212620408));
#24876=CARTESIAN_POINT('Ctrl Pts',(0.0344244045173309,-0.411552957311693,
1.706752));
#24877=CARTESIAN_POINT('Ctrl Pts',(-0.0344244045173315,-0.411552957311693,
1.706752));
#24878=CARTESIAN_POINT('Ctrl Pts',(-0.0717778861362658,-0.407041111792943,
1.70562212620408));
#24879=CARTESIAN_POINT('Ctrl Pts',(-0.143648558862932,-0.387888272594439,
1.70107730356824));
#24880=CARTESIAN_POINT('Ctrl Pts',(-0.178166559972325,-0.373243761060364,
1.69769003172132));
#24881=CARTESIAN_POINT('Ctrl Pts',(-0.244262842368624,-0.335108247315849,
1.68958170688653));
#24882=CARTESIAN_POINT('Ctrl Pts',(-0.283214707341173,-0.303141259068212,
1.68332504372461));
#24883=CARTESIAN_POINT('Ctrl Pts',(-0.341837165343982,-0.236152929235937,
1.67246562047521));
#24884=CARTESIAN_POINT('Ctrl Pts',(-0.368536561654408,-0.192480977588835,
1.66658649961961));
#24885=CARTESIAN_POINT('Ctrl Pts',(-0.394174530911059,-0.123823518623745,
1.66063136041479));
#24886=CARTESIAN_POINT('Ctrl Pts',(-0.400393769631748,-0.101649918886749,
1.65912839404491));
#24887=CARTESIAN_POINT('Ctrl Pts',(-0.404717578595297,-0.0793800000000001,
1.65807299932179));
#24888=CARTESIAN_POINT('',(-0.886256117232624,-0.07938,1.45861320581289));
#24889=CARTESIAN_POINT('Origin',(0.,-0.07938,0.));
#24890=CARTESIAN_POINT('',(-1.45861320581289,-0.07938,0.886256117232623));
#24891=CARTESIAN_POINT('Ctrl Pts',(-0.886256117232623,-0.0793800000000001,
1.45861320581289));
#24892=CARTESIAN_POINT('Ctrl Pts',(-0.890059788636852,-0.101649918886749,
1.45630208793976));
#24893=CARTESIAN_POINT('Ctrl Pts',(-0.895520212222106,-0.123823518623745,
1.45296717977858));
#24894=CARTESIAN_POINT('Ctrl Pts',(-0.917859913453974,-0.192480977588835,
1.43904931717599));
#24895=CARTESIAN_POINT('Ctrl Pts',(-0.940896403863071,-0.236152929235937,
1.4243271592157));
#24896=CARTESIAN_POINT('Ctrl Pts',(-0.990027513266105,-0.303141259068211,
1.39055359345152));
#24897=CARTESIAN_POINT('Ctrl Pts',(-1.02199477007745,-0.335108247315848,
1.36743459453896));
#24898=CARTESIAN_POINT('Ctrl Pts',(-1.07446535104584,-0.373243761060364,
1.32643091652006));
#24899=CARTESIAN_POINT('Ctrl Pts',(-1.10126842659597,-0.387888272594439,
1.30441816675528));
#24900=CARTESIAN_POINT('Ctrl Pts',(-1.15530234155453,-0.407041111792943,
1.25681160160691));
#24901=CARTESIAN_POINT('Ctrl Pts',(-1.18251418313119,-0.411552957311693,
1.23119764287622));
#24902=CARTESIAN_POINT('Ctrl Pts',(-1.23119764287622,-0.411552957311693,
1.18251418313119));
#24903=CARTESIAN_POINT('Ctrl Pts',(-1.25681160160691,-0.407041111792943,
1.15530234155453));
#24904=CARTESIAN_POINT('Ctrl Pts',(-1.30441816675528,-0.387888272594439,
1.10126842659597));
#24905=CARTESIAN_POINT('Ctrl Pts',(-1.32643091652006,-0.373243761060365,
1.07446535104584));
#24906=CARTESIAN_POINT('Ctrl Pts',(-1.36743459453896,-0.335108247315849,
1.02199477007745));
#24907=CARTESIAN_POINT('Ctrl Pts',(-1.39055359345152,-0.303141259068212,
0.990027513266106));
#24908=CARTESIAN_POINT('Ctrl Pts',(-1.4243271592157,-0.236152929235938,
0.940896403863071));
#24909=CARTESIAN_POINT('Ctrl Pts',(-1.43904931717599,-0.192480977588836,
0.917859913453974));
#24910=CARTESIAN_POINT('Ctrl Pts',(-1.45296717977858,-0.123823518623746,
0.895520212222106));
#24911=CARTESIAN_POINT('Ctrl Pts',(-1.45630208793976,-0.101649918886749,
0.890059788636852));
#24912=CARTESIAN_POINT('Ctrl Pts',(-1.45861320581289,-0.0793800000000001,
0.886256117232623));
#24913=CARTESIAN_POINT('',(-1.65807299932179,-0.07938,0.404717578595295));
#24914=CARTESIAN_POINT('Origin',(0.,-0.07938,0.));
#24915=CARTESIAN_POINT('',(-1.706752,-0.411552957311693,2.08591827245526E-16));
#24916=CARTESIAN_POINT('Ctrl Pts',(-1.65807299932179,-0.0793800000000001,
0.404717578595296));
#24917=CARTESIAN_POINT('Ctrl Pts',(-1.65912839404491,-0.101649918886749,
0.400393769631747));
#24918=CARTESIAN_POINT('Ctrl Pts',(-1.66063136041479,-0.123823518623745,
0.394174530911058));
#24919=CARTESIAN_POINT('Ctrl Pts',(-1.66658649961961,-0.192480977588835,
0.368536561654407));
#24920=CARTESIAN_POINT('Ctrl Pts',(-1.67246562047521,-0.236152929235937,
0.341837165343982));
#24921=CARTESIAN_POINT('Ctrl Pts',(-1.68332504372461,-0.303141259068211,
0.283214707341173));
#24922=CARTESIAN_POINT('Ctrl Pts',(-1.68958170688653,-0.335108247315848,
0.244262842368623));
#24923=CARTESIAN_POINT('Ctrl Pts',(-1.69769003172132,-0.373243761060364,
0.178166559972324));
#24924=CARTESIAN_POINT('Ctrl Pts',(-1.70107730356824,-0.387888272594439,
0.143648558862931));
#24925=CARTESIAN_POINT('Ctrl Pts',(-1.70562212620408,-0.407041111792943,
0.0717778861362656));
#24926=CARTESIAN_POINT('Ctrl Pts',(-1.706752,-0.411552957311693,0.0344244045173313));
#24927=CARTESIAN_POINT('Ctrl Pts',(-1.706752,-0.411552957311693,2.08166817117217E-16));
#24928=CARTESIAN_POINT('',(-1.706752,-0.47628,2.09016837373834E-16));
#24929=CARTESIAN_POINT('',(-1.706752,-0.27783,2.09016837373834E-16));
#24930=CARTESIAN_POINT('Origin',(0.,-0.47628,0.));
#24931=CARTESIAN_POINT('',(-1.65807299932179,-0.07938,-0.404717578595296));
#24932=CARTESIAN_POINT('Ctrl Pts',(-1.706752,-0.411552957311693,2.0122792321331E-16));
#24933=CARTESIAN_POINT('Ctrl Pts',(-1.706752,-0.411552957311693,-0.0344244045173309));
#24934=CARTESIAN_POINT('Ctrl Pts',(-1.70562212620408,-0.407041111792943,
-0.0717778861362652));
#24935=CARTESIAN_POINT('Ctrl Pts',(-1.70107730356824,-0.387888272594439,
-0.143648558862931));
#24936=CARTESIAN_POINT('Ctrl Pts',(-1.69769003172132,-0.373243761060365,
-0.178166559972324));
#24937=CARTESIAN_POINT('Ctrl Pts',(-1.68958170688653,-0.335108247315849,
-0.244262842368623));
#24938=CARTESIAN_POINT('Ctrl Pts',(-1.68332504372461,-0.303141259068212,
-0.283214707341173));
#24939=CARTESIAN_POINT('Ctrl Pts',(-1.67246562047521,-0.236152929235938,
-0.341837165343982));
#24940=CARTESIAN_POINT('Ctrl Pts',(-1.66658649961961,-0.192480977588836,
-0.368536561654407));
#24941=CARTESIAN_POINT('Ctrl Pts',(-1.66063136041479,-0.123823518623745,
-0.394174530911059));
#24942=CARTESIAN_POINT('Ctrl Pts',(-1.65912839404491,-0.101649918886749,
-0.400393769631748));
#24943=CARTESIAN_POINT('Ctrl Pts',(-1.65807299932179,-0.0793800000000001,
-0.404717578595296));
#24944=CARTESIAN_POINT('',(-1.45861320581289,-0.07938,-0.886256117232623));
#24945=CARTESIAN_POINT('Origin',(0.,-0.07938,0.));
#24946=CARTESIAN_POINT('',(-0.886256117232623,-0.07938,-1.45861320581289));
#24947=CARTESIAN_POINT('Ctrl Pts',(-1.45861320581289,-0.0793800000000001,
-0.886256117232623));
#24948=CARTESIAN_POINT('Ctrl Pts',(-1.45630208793976,-0.101649918886749,
-0.890059788636852));
#24949=CARTESIAN_POINT('Ctrl Pts',(-1.45296717977858,-0.123823518623745,
-0.895520212222106));
#24950=CARTESIAN_POINT('Ctrl Pts',(-1.43904931717599,-0.192480977588835,
-0.917859913453974));
#24951=CARTESIAN_POINT('Ctrl Pts',(-1.4243271592157,-0.236152929235937,
-0.940896403863072));
#24952=CARTESIAN_POINT('Ctrl Pts',(-1.39055359345152,-0.303141259068212,
-0.990027513266106));
#24953=CARTESIAN_POINT('Ctrl Pts',(-1.36743459453896,-0.335108247315849,
-1.02199477007745));
#24954=CARTESIAN_POINT('Ctrl Pts',(-1.32643091652006,-0.373243761060364,
-1.07446535104584));
#24955=CARTESIAN_POINT('Ctrl Pts',(-1.30441816675528,-0.387888272594439,
-1.10126842659597));
#24956=CARTESIAN_POINT('Ctrl Pts',(-1.25681160160691,-0.407041111792943,
-1.15530234155453));
#24957=CARTESIAN_POINT('Ctrl Pts',(-1.23119764287622,-0.411552957311693,
-1.18251418313119));
#24958=CARTESIAN_POINT('Ctrl Pts',(-1.18251418313119,-0.411552957311693,
-1.23119764287622));
#24959=CARTESIAN_POINT('Ctrl Pts',(-1.15530234155453,-0.407041111792943,
-1.25681160160691));
#24960=CARTESIAN_POINT('Ctrl Pts',(-1.10126842659597,-0.387888272594439,
-1.30441816675528));
#24961=CARTESIAN_POINT('Ctrl Pts',(-1.07446535104584,-0.373243761060364,
-1.32643091652006));
#24962=CARTESIAN_POINT('Ctrl Pts',(-1.02199477007745,-0.335108247315848,
-1.36743459453896));
#24963=CARTESIAN_POINT('Ctrl Pts',(-0.990027513266105,-0.303141259068211,
-1.39055359345152));
#24964=CARTESIAN_POINT('Ctrl Pts',(-0.940896403863071,-0.236152929235936,
-1.42432715921571));
#24965=CARTESIAN_POINT('Ctrl Pts',(-0.917859913453974,-0.192480977588835,
-1.43904931717599));
#24966=CARTESIAN_POINT('Ctrl Pts',(-0.895520212222106,-0.123823518623745,
-1.45296717977858));
#24967=CARTESIAN_POINT('Ctrl Pts',(-0.890059788636851,-0.101649918886749,
-1.45630208793976));
#24968=CARTESIAN_POINT('Ctrl Pts',(-0.886256117232623,-0.0793800000000001,
-1.45861320581289));
#24969=CARTESIAN_POINT('',(-0.404717578595295,-0.07938,-1.65807299932179));
#24970=CARTESIAN_POINT('Origin',(0.,-0.07938,0.));
#24971=CARTESIAN_POINT('',(0.404717578595296,-0.07938,-1.65807299932179));
#24972=CARTESIAN_POINT('Ctrl Pts',(-0.404717578595296,-0.0793800000000001,
-1.65807299932179));
#24973=CARTESIAN_POINT('Ctrl Pts',(-0.400393769631747,-0.101649918886749,
-1.65912839404491));
#24974=CARTESIAN_POINT('Ctrl Pts',(-0.394174530911058,-0.123823518623746,
-1.66063136041479));
#24975=CARTESIAN_POINT('Ctrl Pts',(-0.368536561654407,-0.192480977588836,
-1.66658649961961));
#24976=CARTESIAN_POINT('Ctrl Pts',(-0.341837165343982,-0.236152929235938,
-1.67246562047521));
#24977=CARTESIAN_POINT('Ctrl Pts',(-0.283214707341173,-0.303141259068212,
-1.68332504372461));
#24978=CARTESIAN_POINT('Ctrl Pts',(-0.244262842368623,-0.335108247315849,
-1.68958170688653));
#24979=CARTESIAN_POINT('Ctrl Pts',(-0.178166559972324,-0.373243761060364,
-1.69769003172132));
#24980=CARTESIAN_POINT('Ctrl Pts',(-0.143648558862931,-0.387888272594439,
-1.70107730356824));
#24981=CARTESIAN_POINT('Ctrl Pts',(-0.0717778861362653,-0.407041111792943,
-1.70562212620408));
#24982=CARTESIAN_POINT('Ctrl Pts',(-0.034424404517331,-0.411552957311693,
-1.706752));
#24983=CARTESIAN_POINT('Ctrl Pts',(0.0344244045173312,-0.411552957311693,
-1.706752));
#24984=CARTESIAN_POINT('Ctrl Pts',(0.0717778861362655,-0.407041111792943,
-1.70562212620408));
#24985=CARTESIAN_POINT('Ctrl Pts',(0.143648558862931,-0.387888272594439,
-1.70107730356824));
#24986=CARTESIAN_POINT('Ctrl Pts',(0.178166559972324,-0.373243761060364,
-1.69769003172132));
#24987=CARTESIAN_POINT('Ctrl Pts',(0.244262842368623,-0.335108247315849,
-1.68958170688653));
#24988=CARTESIAN_POINT('Ctrl Pts',(0.283214707341173,-0.303141259068212,
-1.68332504372461));
#24989=CARTESIAN_POINT('Ctrl Pts',(0.341837165343982,-0.236152929235937,
-1.67246562047521));
#24990=CARTESIAN_POINT('Ctrl Pts',(0.368536561654407,-0.192480977588835,
-1.66658649961961));
#24991=CARTESIAN_POINT('Ctrl Pts',(0.394174530911059,-0.123823518623745,
-1.66063136041479));
#24992=CARTESIAN_POINT('Ctrl Pts',(0.400393769631748,-0.101649918886749,
-1.65912839404491));
#24993=CARTESIAN_POINT('Ctrl Pts',(0.404717578595296,-0.0793800000000001,
-1.65807299932179));
#24994=CARTESIAN_POINT('',(0.886256117232623,-0.07938,-1.45861320581289));
#24995=CARTESIAN_POINT('Origin',(0.,-0.07938,0.));
#24996=CARTESIAN_POINT('',(1.45861320581289,-0.07938,-0.886256117232623));
#24997=CARTESIAN_POINT('Ctrl Pts',(0.886256117232623,-0.0793800000000001,
-1.45861320581289));
#24998=CARTESIAN_POINT('Ctrl Pts',(0.890059788636852,-0.101649918886749,
-1.45630208793976));
#24999=CARTESIAN_POINT('Ctrl Pts',(0.895520212222106,-0.123823518623745,
-1.45296717977858));
#25000=CARTESIAN_POINT('Ctrl Pts',(0.917859913453974,-0.192480977588835,
-1.43904931717599));
#25001=CARTESIAN_POINT('Ctrl Pts',(0.940896403863072,-0.236152929235937,
-1.4243271592157));
#25002=CARTESIAN_POINT('Ctrl Pts',(0.990027513266106,-0.303141259068211,
-1.39055359345152));
#25003=CARTESIAN_POINT('Ctrl Pts',(1.02199477007745,-0.335108247315849,
-1.36743459453896));
#25004=CARTESIAN_POINT('Ctrl Pts',(1.07446535104584,-0.373243761060364,
-1.32643091652006));
#25005=CARTESIAN_POINT('Ctrl Pts',(1.10126842659597,-0.387888272594439,
-1.30441816675528));
#25006=CARTESIAN_POINT('Ctrl Pts',(1.15530234155453,-0.407041111792943,
-1.25681160160691));
#25007=CARTESIAN_POINT('Ctrl Pts',(1.18251418313119,-0.411552957311693,
-1.23119764287622));
#25008=CARTESIAN_POINT('Ctrl Pts',(1.23119764287622,-0.411552957311693,
-1.18251418313119));
#25009=CARTESIAN_POINT('Ctrl Pts',(1.25681160160691,-0.407041111792943,
-1.15530234155453));
#25010=CARTESIAN_POINT('Ctrl Pts',(1.30441816675528,-0.387888272594439,
-1.10126842659597));
#25011=CARTESIAN_POINT('Ctrl Pts',(1.32643091652006,-0.373243761060364,
-1.07446535104584));
#25012=CARTESIAN_POINT('Ctrl Pts',(1.36743459453896,-0.335108247315849,
-1.02199477007745));
#25013=CARTESIAN_POINT('Ctrl Pts',(1.39055359345152,-0.303141259068212,
-0.990027513266105));
#25014=CARTESIAN_POINT('Ctrl Pts',(1.4243271592157,-0.236152929235937,-0.940896403863071));
#25015=CARTESIAN_POINT('Ctrl Pts',(1.43904931717599,-0.192480977588835,
-0.917859913453974));
#25016=CARTESIAN_POINT('Ctrl Pts',(1.45296717977858,-0.123823518623745,
-0.895520212222106));
#25017=CARTESIAN_POINT('Ctrl Pts',(1.45630208793976,-0.101649918886749,
-0.890059788636852));
#25018=CARTESIAN_POINT('Ctrl Pts',(1.45861320581289,-0.0793800000000001,
-0.886256117232623));
#25019=CARTESIAN_POINT('',(1.65807299932179,-0.07938,-0.404717578595296));
#25020=CARTESIAN_POINT('Origin',(0.,-0.07938,0.));
#25021=CARTESIAN_POINT('',(1.65807299932179,-0.07938,0.404717578595296));
#25022=CARTESIAN_POINT('Ctrl Pts',(1.65807299932179,-0.0793800000000001,
-0.404717578595296));
#25023=CARTESIAN_POINT('Ctrl Pts',(1.65912839404491,-0.101649918886749,
-0.400393769631747));
#25024=CARTESIAN_POINT('Ctrl Pts',(1.66063136041479,-0.123823518623745,
-0.394174530911058));
#25025=CARTESIAN_POINT('Ctrl Pts',(1.66658649961961,-0.192480977588835,
-0.368536561654407));
#25026=CARTESIAN_POINT('Ctrl Pts',(1.67246562047521,-0.236152929235937,
-0.341837165343982));
#25027=CARTESIAN_POINT('Ctrl Pts',(1.68332504372461,-0.303141259068212,
-0.283214707341173));
#25028=CARTESIAN_POINT('Ctrl Pts',(1.68958170688653,-0.335108247315849,
-0.244262842368623));
#25029=CARTESIAN_POINT('Ctrl Pts',(1.69769003172132,-0.373243761060364,
-0.178166559972324));
#25030=CARTESIAN_POINT('Ctrl Pts',(1.70107730356824,-0.387888272594439,
-0.143648558862931));
#25031=CARTESIAN_POINT('Ctrl Pts',(1.70562212620408,-0.407041111792943,
-0.0717778861362655));
#25032=CARTESIAN_POINT('Ctrl Pts',(1.706752,-0.411552957311693,-0.0344244045173312));
#25033=CARTESIAN_POINT('Ctrl Pts',(1.706752,-0.411552957311693,0.0344244045173312));
#25034=CARTESIAN_POINT('Ctrl Pts',(1.70562212620408,-0.407041111792943,
0.0717778861362655));
#25035=CARTESIAN_POINT('Ctrl Pts',(1.70107730356824,-0.387888272594439,
0.143648558862931));
#25036=CARTESIAN_POINT('Ctrl Pts',(1.69769003172132,-0.373243761060364,
0.178166559972324));
#25037=CARTESIAN_POINT('Ctrl Pts',(1.68958170688653,-0.335108247315849,
0.244262842368623));
#25038=CARTESIAN_POINT('Ctrl Pts',(1.68332504372461,-0.303141259068212,
0.283214707341173));
#25039=CARTESIAN_POINT('Ctrl Pts',(1.67246562047521,-0.236152929235937,
0.341837165343982));
#25040=CARTESIAN_POINT('Ctrl Pts',(1.66658649961961,-0.192480977588835,
0.368536561654407));
#25041=CARTESIAN_POINT('Ctrl Pts',(1.66063136041479,-0.123823518623745,
0.394174530911058));
#25042=CARTESIAN_POINT('Ctrl Pts',(1.65912839404491,-0.101649918886749,
0.400393769631747));
#25043=CARTESIAN_POINT('Ctrl Pts',(1.65807299932179,-0.0793800000000001,
0.404717578595296));
#25044=CARTESIAN_POINT('Origin',(0.,-0.07938,0.));
#25045=CARTESIAN_POINT('Origin',(0.,-0.07938,0.));
#25046=CARTESIAN_POINT('',(0.397005914195118,-0.07938,1.59456899932179));
#25047=CARTESIAN_POINT('Origin',(0.,-0.07938,0.));
#25048=CARTESIAN_POINT('Origin',(-3.33066907387547E-16,-0.07938,1.675));
#25049=CARTESIAN_POINT('Origin',(-3.33066907387547E-16,0.,1.675));
#25050=CARTESIAN_POINT('',(-0.397005914195118,-0.07938,1.59456899932179));
#25051=CARTESIAN_POINT('Ctrl Pts',(-0.397005914195119,-0.0793800000000001,
1.59456899932179));
#25052=CARTESIAN_POINT('Ctrl Pts',(-0.3886265584581,-0.123401821157026,
1.59665523941937));
#25053=CARTESIAN_POINT('Ctrl Pts',(-0.373030350867485,-0.166543350814306,
1.60050712143809));
#25054=CARTESIAN_POINT('Ctrl Pts',(-0.333298652394954,-0.237231147975234,
1.60919314384089));
#25055=CARTESIAN_POINT('Ctrl Pts',(-0.311480544243687,-0.266264900654909,
1.61365775139403));
#25056=CARTESIAN_POINT('Ctrl Pts',(-0.261368388670537,-0.317195968905306,
1.62252828437015));
#25057=CARTESIAN_POINT('Ctrl Pts',(-0.233069203882014,-0.33909093068465,
1.62691869420078));
#25058=CARTESIAN_POINT('Ctrl Pts',(-0.174042761838764,-0.373586846396559,
1.63426473152765));
#25059=CARTESIAN_POINT('Ctrl Pts',(-0.14036578147155,-0.388086240756494,
1.63761964365402));
#25060=CARTESIAN_POINT('Ctrl Pts',(-0.0701778381840615,-0.407068917407805,
1.64212536811722));
#25061=CARTESIAN_POINT('Ctrl Pts',(-0.0336652739555918,-0.411552957311693,
1.643248));
#25062=CARTESIAN_POINT('Ctrl Pts',(0.0336652739555913,-0.411552957311693,
1.643248));
#25063=CARTESIAN_POINT('Ctrl Pts',(0.070177838184061,-0.407068917407805,
1.64212536811722));
#25064=CARTESIAN_POINT('Ctrl Pts',(0.140365781471549,-0.388086240756494,
1.63761964365402));
#25065=CARTESIAN_POINT('Ctrl Pts',(0.174042761838763,-0.373586846396559,
1.63426473152765));
#25066=CARTESIAN_POINT('Ctrl Pts',(0.233069203882014,-0.33909093068465,
1.62691869420078));
#25067=CARTESIAN_POINT('Ctrl Pts',(0.261368388670536,-0.317195968905306,
1.62252828437015));
#25068=CARTESIAN_POINT('Ctrl Pts',(0.311480544243686,-0.266264900654908,
1.61365775139403));
#25069=CARTESIAN_POINT('Ctrl Pts',(0.333298652394954,-0.237231147975234,
1.60919314384089));
#25070=CARTESIAN_POINT('Ctrl Pts',(0.373030350867484,-0.166543350814306,
1.60050712143809));
#25071=CARTESIAN_POINT('Ctrl Pts',(0.388626558458099,-0.123401821157026,
1.59665523941937));
#25072=CARTESIAN_POINT('Ctrl Pts',(0.397005914195118,-0.07938,1.59456899932179));
#25073=CARTESIAN_POINT('Origin',(-3.33066907387547E-16,-0.07938,1.675));
#25074=CARTESIAN_POINT('Origin',(0.,-0.07938,0.));
#25075=CARTESIAN_POINT('',(-0.846804978391754,-0.07938,1.40825612658882));
#25076=CARTESIAN_POINT('Origin',(0.,-0.07938,0.));
#25077=CARTESIAN_POINT('Origin',(-1.18440385848747,-0.07938,1.18440385848747));
#25078=CARTESIAN_POINT('Origin',(-1.18440385848747,0.,1.18440385848747));
#25079=CARTESIAN_POINT('',(-1.40825612658882,-0.07938,0.846804978391753));
#25080=CARTESIAN_POINT('Ctrl Pts',(-1.40825612658882,-0.0793800000000001,
0.846804978391753));
#25081=CARTESIAN_POINT('Ctrl Pts',(-1.40380622184538,-0.123401821157026,
0.854205272175555));
#25082=CARTESIAN_POINT('Ctrl Pts',(-1.39550172959303,-0.166543350814306,
0.867957148219442));
#25083=CARTESIAN_POINT('Ctrl Pts',(-1.3735491215176,-0.237231147975235,
0.902193646979983));
#25084=CARTESIAN_POINT('Ctrl Pts',(-1.36127834356734,-0.266264900654909,
0.920778333482565));
#25085=CARTESIAN_POINT('Ctrl Pts',(-1.33211611256184,-0.317195968905306,
0.962485392528369));
#25086=CARTESIAN_POINT('Ctrl Pts',(-1.31521005565926,-0.339090930684651,
0.985600426557816));
#25087=CARTESIAN_POINT('Ctrl Pts',(-1.27866649102984,-0.373586846396559,
1.03253285680459));
#25088=CARTESIAN_POINT('Ctrl Pts',(-1.25722555095714,-0.388086240756494,
1.05871835910697));
#25089=CARTESIAN_POINT('Ctrl Pts',(-1.2107812086231,-0.407068917407805,
1.11153475808518));
#25090=CARTESIAN_POINT('Ctrl Pts',(-1.18575674747573,-0.411552957311693,
1.13814686046673));
#25091=CARTESIAN_POINT('Ctrl Pts',(-1.13814686046673,-0.411552957311693,
1.18575674747573));
#25092=CARTESIAN_POINT('Ctrl Pts',(-1.11153475808518,-0.407068917407805,
1.2107812086231));
#25093=CARTESIAN_POINT('Ctrl Pts',(-1.05871835910697,-0.388086240756494,
1.25722555095714));
#25094=CARTESIAN_POINT('Ctrl Pts',(-1.03253285680459,-0.373586846396559,
1.27866649102984));
#25095=CARTESIAN_POINT('Ctrl Pts',(-0.985600426557816,-0.33909093068465,
1.31521005565926));
#25096=CARTESIAN_POINT('Ctrl Pts',(-0.962485392528369,-0.317195968905306,
1.33211611256184));
#25097=CARTESIAN_POINT('Ctrl Pts',(-0.920778333482565,-0.266264900654908,
1.36127834356734));
#25098=CARTESIAN_POINT('Ctrl Pts',(-0.902193646979983,-0.237231147975234,
1.3735491215176));
#25099=CARTESIAN_POINT('Ctrl Pts',(-0.867957148219442,-0.166543350814306,
1.39550172959303));
#25100=CARTESIAN_POINT('Ctrl Pts',(-0.854205272175555,-0.123401821157026,
1.40380622184538));
#25101=CARTESIAN_POINT('Ctrl Pts',(-0.846804978391753,-0.0793800000000001,
1.40825612658882));
#25102=CARTESIAN_POINT('Origin',(-1.18440385848747,-0.07938,1.18440385848747));
#25103=CARTESIAN_POINT('Origin',(0.,-0.07938,0.));
#25104=CARTESIAN_POINT('',(-1.59456899932179,-0.07938,0.397005914195118));
#25105=CARTESIAN_POINT('Origin',(0.,-0.07938,0.));
#25106=CARTESIAN_POINT('Origin',(-1.675,-0.07938,-2.22044604925031E-16));
#25107=CARTESIAN_POINT('Origin',(-1.675,0.,-2.22044604925031E-16));
#25108=CARTESIAN_POINT('',(-1.59456899932179,-0.07938,-0.397005914195118));
#25109=CARTESIAN_POINT('',(-1.643248,-0.411552957311693,3.47540551556327E-18));
#25110=CARTESIAN_POINT('Ctrl Pts',(-1.59456899932179,-0.0793800000000001,
-0.397005914195119));
#25111=CARTESIAN_POINT('Ctrl Pts',(-1.59665523941937,-0.123401821157026,
-0.388626558458099));
#25112=CARTESIAN_POINT('Ctrl Pts',(-1.60050712143809,-0.166543350814306,
-0.373030350867485));
#25113=CARTESIAN_POINT('Ctrl Pts',(-1.60919314384089,-0.237231147975234,
-0.333298652394954));
#25114=CARTESIAN_POINT('Ctrl Pts',(-1.61365775139403,-0.266264900654909,
-0.311480544243686));
#25115=CARTESIAN_POINT('Ctrl Pts',(-1.62252828437015,-0.317195968905306,
-0.261368388670537));
#25116=CARTESIAN_POINT('Ctrl Pts',(-1.62691869420078,-0.33909093068465,
-0.233069203882014));
#25117=CARTESIAN_POINT('Ctrl Pts',(-1.63426473152765,-0.373586846396559,
-0.174042761838764));
#25118=CARTESIAN_POINT('Ctrl Pts',(-1.63761964365402,-0.388086240756494,
-0.140365781471549));
#25119=CARTESIAN_POINT('Ctrl Pts',(-1.64212536811722,-0.407068917407805,
-0.0701778381840614));
#25120=CARTESIAN_POINT('Ctrl Pts',(-1.643248,-0.411552957311693,-0.0336652739555917));
#25121=CARTESIAN_POINT('Ctrl Pts',(-1.643248,-0.411552957311693,-2.0122792321331E-16));
#25122=CARTESIAN_POINT('Origin',(-1.675,-0.07938,-2.22044604925031E-16));
#25123=CARTESIAN_POINT('Ctrl Pts',(-1.643248,-0.411552957311693,-1.94289029309402E-16));
#25124=CARTESIAN_POINT('Ctrl Pts',(-1.643248,-0.411552957311693,0.0336652739555913));
#25125=CARTESIAN_POINT('Ctrl Pts',(-1.64212536811722,-0.407068917407805,
0.0701778381840609));
#25126=CARTESIAN_POINT('Ctrl Pts',(-1.63761964365402,-0.388086240756494,
0.140365781471549));
#25127=CARTESIAN_POINT('Ctrl Pts',(-1.63426473152765,-0.373586846396559,
0.174042761838763));
#25128=CARTESIAN_POINT('Ctrl Pts',(-1.62691869420078,-0.33909093068465,
0.233069203882014));
#25129=CARTESIAN_POINT('Ctrl Pts',(-1.62252828437015,-0.317195968905306,
0.261368388670536));
#25130=CARTESIAN_POINT('Ctrl Pts',(-1.61365775139403,-0.266264900654909,
0.311480544243686));
#25131=CARTESIAN_POINT('Ctrl Pts',(-1.60919314384089,-0.237231147975235,
0.333298652394954));
#25132=CARTESIAN_POINT('Ctrl Pts',(-1.60050712143809,-0.166543350814306,
0.373030350867484));
#25133=CARTESIAN_POINT('Ctrl Pts',(-1.59665523941937,-0.123401821157026,
0.388626558458099));
#25134=CARTESIAN_POINT('Ctrl Pts',(-1.59456899932179,-0.0793800000000001,
0.397005914195118));
#25135=CARTESIAN_POINT('Origin',(0.,-0.07938,0.));
#25136=CARTESIAN_POINT('',(-1.40825612658882,-0.07938,-0.846804978391753));
#25137=CARTESIAN_POINT('Origin',(0.,-0.07938,0.));
#25138=CARTESIAN_POINT('Origin',(-1.18440385848747,-0.07938,-1.18440385848747));
#25139=CARTESIAN_POINT('Origin',(-1.18440385848747,0.,-1.18440385848747));
#25140=CARTESIAN_POINT('',(-0.846804978391753,-0.07938,-1.40825612658882));
#25141=CARTESIAN_POINT('Ctrl Pts',(-0.846804978391753,-0.0793800000000001,
-1.40825612658882));
#25142=CARTESIAN_POINT('Ctrl Pts',(-0.854205272175555,-0.123401821157026,
-1.40380622184538));
#25143=CARTESIAN_POINT('Ctrl Pts',(-0.867957148219442,-0.166543350814306,
-1.39550172959303));
#25144=CARTESIAN_POINT('Ctrl Pts',(-0.902193646979982,-0.237231147975234,
-1.3735491215176));
#25145=CARTESIAN_POINT('Ctrl Pts',(-0.920778333482564,-0.266264900654908,
-1.36127834356734));
#25146=CARTESIAN_POINT('Ctrl Pts',(-0.962485392528368,-0.317195968905306,
-1.33211611256184));
#25147=CARTESIAN_POINT('Ctrl Pts',(-0.985600426557816,-0.33909093068465,
-1.31521005565926));
#25148=CARTESIAN_POINT('Ctrl Pts',(-1.03253285680459,-0.373586846396559,
-1.27866649102984));
#25149=CARTESIAN_POINT('Ctrl Pts',(-1.05871835910697,-0.388086240756494,
-1.25722555095714));
#25150=CARTESIAN_POINT('Ctrl Pts',(-1.11153475808518,-0.407068917407805,
-1.2107812086231));
#25151=CARTESIAN_POINT('Ctrl Pts',(-1.13814686046673,-0.411552957311693,
-1.18575674747573));
#25152=CARTESIAN_POINT('Ctrl Pts',(-1.18575674747573,-0.411552957311693,
-1.13814686046673));
#25153=CARTESIAN_POINT('Ctrl Pts',(-1.2107812086231,-0.407068917407805,
-1.11153475808518));
#25154=CARTESIAN_POINT('Ctrl Pts',(-1.25722555095714,-0.388086240756494,
-1.05871835910697));
#25155=CARTESIAN_POINT('Ctrl Pts',(-1.27866649102984,-0.373586846396559,
-1.03253285680459));
#25156=CARTESIAN_POINT('Ctrl Pts',(-1.31521005565926,-0.33909093068465,
-0.985600426557816));
#25157=CARTESIAN_POINT('Ctrl Pts',(-1.33211611256184,-0.317195968905306,
-0.962485392528369));
#25158=CARTESIAN_POINT('Ctrl Pts',(-1.36127834356734,-0.266264900654909,
-0.920778333482565));
#25159=CARTESIAN_POINT('Ctrl Pts',(-1.3735491215176,-0.237231147975234,
-0.902193646979983));
#25160=CARTESIAN_POINT('Ctrl Pts',(-1.39550172959303,-0.166543350814306,
-0.867957148219442));
#25161=CARTESIAN_POINT('Ctrl Pts',(-1.40380622184538,-0.123401821157026,
-0.854205272175555));
#25162=CARTESIAN_POINT('Ctrl Pts',(-1.40825612658882,-0.07938,-0.846804978391753));
#25163=CARTESIAN_POINT('Origin',(-1.18440385848747,-0.07938,-1.18440385848747));
#25164=CARTESIAN_POINT('Origin',(0.,-0.07938,0.));
#25165=CARTESIAN_POINT('',(-0.397005914195118,-0.07938,-1.59456899932179));
#25166=CARTESIAN_POINT('Origin',(0.,-0.07938,0.));
#25167=CARTESIAN_POINT('Origin',(1.11022302462516E-16,-0.07938,-1.675));
#25168=CARTESIAN_POINT('Origin',(1.11022302462516E-16,0.,-1.675));
#25169=CARTESIAN_POINT('',(0.397005914195118,-0.07938,-1.59456899932179));
#25170=CARTESIAN_POINT('Ctrl Pts',(0.397005914195119,-0.0793800000000001,
-1.59456899932179));
#25171=CARTESIAN_POINT('Ctrl Pts',(0.388626558458099,-0.123401821157026,
-1.59665523941937));
#25172=CARTESIAN_POINT('Ctrl Pts',(0.373030350867485,-0.166543350814306,
-1.60050712143809));
#25173=CARTESIAN_POINT('Ctrl Pts',(0.333298652394954,-0.237231147975234,
-1.60919314384089));
#25174=CARTESIAN_POINT('Ctrl Pts',(0.311480544243686,-0.266264900654909,
-1.61365775139403));
#25175=CARTESIAN_POINT('Ctrl Pts',(0.261368388670537,-0.317195968905306,
-1.62252828437015));
#25176=CARTESIAN_POINT('Ctrl Pts',(0.233069203882014,-0.33909093068465,
-1.62691869420078));
#25177=CARTESIAN_POINT('Ctrl Pts',(0.174042761838763,-0.373586846396559,
-1.63426473152765));
#25178=CARTESIAN_POINT('Ctrl Pts',(0.140365781471549,-0.388086240756494,
-1.63761964365402));
#25179=CARTESIAN_POINT('Ctrl Pts',(0.0701778381840612,-0.407068917407805,
-1.64212536811722));
#25180=CARTESIAN_POINT('Ctrl Pts',(0.0336652739555916,-0.411552957311693,
-1.643248));
#25181=CARTESIAN_POINT('Ctrl Pts',(-0.0336652739555915,-0.411552957311693,
-1.643248));
#25182=CARTESIAN_POINT('Ctrl Pts',(-0.0701778381840612,-0.407068917407805,
-1.64212536811722));
#25183=CARTESIAN_POINT('Ctrl Pts',(-0.140365781471549,-0.388086240756494,
-1.63761964365402));
#25184=CARTESIAN_POINT('Ctrl Pts',(-0.174042761838764,-0.373586846396559,
-1.63426473152765));
#25185=CARTESIAN_POINT('Ctrl Pts',(-0.233069203882014,-0.33909093068465,
-1.62691869420078));
#25186=CARTESIAN_POINT('Ctrl Pts',(-0.261368388670536,-0.317195968905306,
-1.62252828437015));
#25187=CARTESIAN_POINT('Ctrl Pts',(-0.311480544243686,-0.266264900654908,
-1.61365775139403));
#25188=CARTESIAN_POINT('Ctrl Pts',(-0.333298652394954,-0.237231147975234,
-1.60919314384089));
#25189=CARTESIAN_POINT('Ctrl Pts',(-0.373030350867485,-0.166543350814306,
-1.60050712143809));
#25190=CARTESIAN_POINT('Ctrl Pts',(-0.388626558458099,-0.123401821157026,
-1.59665523941937));
#25191=CARTESIAN_POINT('Ctrl Pts',(-0.397005914195118,-0.07938,-1.59456899932179));
#25192=CARTESIAN_POINT('Origin',(1.11022302462516E-16,-0.07938,-1.675));
#25193=CARTESIAN_POINT('Origin',(0.,-0.07938,0.));
#25194=CARTESIAN_POINT('',(0.846804978391753,-0.07938,-1.40825612658882));
#25195=CARTESIAN_POINT('Origin',(0.,-0.07938,0.));
#25196=CARTESIAN_POINT('Origin',(1.18440385848747,-0.07938,-1.18440385848747));
#25197=CARTESIAN_POINT('Origin',(1.18440385848747,0.,-1.18440385848747));
#25198=CARTESIAN_POINT('',(1.40825612658882,-0.07938,-0.846804978391753));
#25199=CARTESIAN_POINT('Ctrl Pts',(1.40825612658882,-0.0793800000000001,
-0.846804978391753));
#25200=CARTESIAN_POINT('Ctrl Pts',(1.40380622184538,-0.123401821157026,
-0.854205272175555));
#25201=CARTESIAN_POINT('Ctrl Pts',(1.39550172959303,-0.166543350814306,
-0.867957148219442));
#25202=CARTESIAN_POINT('Ctrl Pts',(1.3735491215176,-0.237231147975234,-0.902193646979983));
#25203=CARTESIAN_POINT('Ctrl Pts',(1.36127834356734,-0.266264900654908,
-0.920778333482565));
#25204=CARTESIAN_POINT('Ctrl Pts',(1.33211611256184,-0.317195968905306,
-0.962485392528369));
#25205=CARTESIAN_POINT('Ctrl Pts',(1.31521005565926,-0.33909093068465,-0.985600426557816));
#25206=CARTESIAN_POINT('Ctrl Pts',(1.27866649102984,-0.373586846396559,
-1.03253285680459));
#25207=CARTESIAN_POINT('Ctrl Pts',(1.25722555095714,-0.388086240756494,
-1.05871835910697));
#25208=CARTESIAN_POINT('Ctrl Pts',(1.2107812086231,-0.407068917407805,-1.11153475808518));
#25209=CARTESIAN_POINT('Ctrl Pts',(1.18575674747573,-0.411552957311693,
-1.13814686046673));
#25210=CARTESIAN_POINT('Ctrl Pts',(1.13814686046673,-0.411552957311693,
-1.18575674747573));
#25211=CARTESIAN_POINT('Ctrl Pts',(1.11153475808518,-0.407068917407805,
-1.2107812086231));
#25212=CARTESIAN_POINT('Ctrl Pts',(1.05871835910697,-0.388086240756494,
-1.25722555095714));
#25213=CARTESIAN_POINT('Ctrl Pts',(1.03253285680459,-0.373586846396559,
-1.27866649102984));
#25214=CARTESIAN_POINT('Ctrl Pts',(0.985600426557816,-0.33909093068465,
-1.31521005565926));
#25215=CARTESIAN_POINT('Ctrl Pts',(0.962485392528369,-0.317195968905306,
-1.33211611256184));
#25216=CARTESIAN_POINT('Ctrl Pts',(0.920778333482565,-0.266264900654909,
-1.36127834356734));
#25217=CARTESIAN_POINT('Ctrl Pts',(0.902193646979983,-0.237231147975234,
-1.3735491215176));
#25218=CARTESIAN_POINT('Ctrl Pts',(0.867957148219442,-0.166543350814306,
-1.39550172959303));
#25219=CARTESIAN_POINT('Ctrl Pts',(0.854205272175555,-0.123401821157026,
-1.40380622184538));
#25220=CARTESIAN_POINT('Ctrl Pts',(0.846804978391753,-0.0793800000000001,
-1.40825612658882));
#25221=CARTESIAN_POINT('Origin',(1.18440385848747,-0.07938,-1.18440385848747));
#25222=CARTESIAN_POINT('Origin',(0.,-0.27783,0.));
#25223=CARTESIAN_POINT('',(-1.643248,-0.47628,2.01239840340529E-16));
#25224=CARTESIAN_POINT('Origin',(0.,-0.47628,0.));
#25225=CARTESIAN_POINT('',(-1.643248,-0.27783,2.01239840340529E-16));
#25226=CARTESIAN_POINT('',(1.59456899932179,-0.07938,0.397005914195118));
#25227=CARTESIAN_POINT('Origin',(0.,-0.07938,0.));
#25228=CARTESIAN_POINT('',(1.59456899932179,-0.07938,-0.397005914195118));
#25229=CARTESIAN_POINT('Ctrl Pts',(1.59456899932179,-0.0793800000000001,
0.397005914195118));
#25230=CARTESIAN_POINT('Ctrl Pts',(1.59665523941937,-0.123401821157026,
0.388626558458099));
#25231=CARTESIAN_POINT('Ctrl Pts',(1.60050712143809,-0.166543350814306,
0.373030350867485));
#25232=CARTESIAN_POINT('Ctrl Pts',(1.60919314384089,-0.237231147975234,
0.333298652394954));
#25233=CARTESIAN_POINT('Ctrl Pts',(1.61365775139403,-0.266264900654909,
0.311480544243686));
#25234=CARTESIAN_POINT('Ctrl Pts',(1.62252828437015,-0.317195968905306,
0.261368388670537));
#25235=CARTESIAN_POINT('Ctrl Pts',(1.62691869420078,-0.33909093068465,0.233069203882014));
#25236=CARTESIAN_POINT('Ctrl Pts',(1.63426473152765,-0.373586846396559,
0.174042761838764));
#25237=CARTESIAN_POINT('Ctrl Pts',(1.63761964365402,-0.388086240756494,
0.140365781471549));
#25238=CARTESIAN_POINT('Ctrl Pts',(1.64212536811722,-0.407068917407805,
0.0701778381840612));
#25239=CARTESIAN_POINT('Ctrl Pts',(1.643248,-0.411552957311693,0.0336652739555916));
#25240=CARTESIAN_POINT('Ctrl Pts',(1.643248,-0.411552957311693,-0.0336652739555916));
#25241=CARTESIAN_POINT('Ctrl Pts',(1.64212536811722,-0.407068917407805,
-0.0701778381840612));
#25242=CARTESIAN_POINT('Ctrl Pts',(1.63761964365402,-0.388086240756494,
-0.140365781471549));
#25243=CARTESIAN_POINT('Ctrl Pts',(1.63426473152765,-0.373586846396559,
-0.174042761838764));
#25244=CARTESIAN_POINT('Ctrl Pts',(1.62691869420078,-0.33909093068465,-0.233069203882014));
#25245=CARTESIAN_POINT('Ctrl Pts',(1.62252828437015,-0.317195968905306,
-0.261368388670537));
#25246=CARTESIAN_POINT('Ctrl Pts',(1.61365775139403,-0.266264900654909,
-0.311480544243686));
#25247=CARTESIAN_POINT('Ctrl Pts',(1.60919314384089,-0.237231147975234,
-0.333298652394954));
#25248=CARTESIAN_POINT('Ctrl Pts',(1.60050712143809,-0.166543350814306,
-0.373030350867485));
#25249=CARTESIAN_POINT('Ctrl Pts',(1.59665523941937,-0.123401821157026,
-0.388626558458099));
#25250=CARTESIAN_POINT('Ctrl Pts',(1.59456899932179,-0.07938,-0.397005914195118));
#25251=CARTESIAN_POINT('Origin',(0.,-0.07938,0.));
#25252=CARTESIAN_POINT('Origin',(0.,-0.07938,0.));
#25253=CARTESIAN_POINT('Origin',(1.675,-0.07938,0.));
#25254=CARTESIAN_POINT('Origin',(1.675,0.,0.));
#25255=CARTESIAN_POINT('Origin',(1.675,-0.07938,0.));
#25256=CARTESIAN_POINT('Origin',(0.,-0.47628,0.));
#25257=CARTESIAN_POINT('Origin',(0.,-0.07938,0.));
#73268=UNCERTAINTY_MEASURE_WITH_UNIT(LENGTH_MEASURE(0.001),#73367,
'DISTANCE_ACCURACY_VALUE',
'Maximum model space distance between geometric entities at asserted c
onnectivities');
#73302=UNCERTAINTY_MEASURE_WITH_UNIT(LENGTH_MEASURE(0.001),#73367,
'DISTANCE_ACCURACY_VALUE',
'Maximum model space distance between geometric entities at asserted c
onnectivities');
#73332=(
GEOMETRIC_REPRESENTATION_CONTEXT(3)
GLOBAL_UNCERTAINTY_ASSIGNED_CONTEXT((#73268))
GLOBAL_UNIT_ASSIGNED_CONTEXT((#73367,#73369,#73370))
REPRESENTATION_CONTEXT('','3D')
);
#73366=(
GEOMETRIC_REPRESENTATION_CONTEXT(3)
GLOBAL_UNCERTAINTY_ASSIGNED_CONTEXT((#73302))
GLOBAL_UNIT_ASSIGNED_CONTEXT((#73367,#73369,#73370))
REPRESENTATION_CONTEXT('','3D')
);
#73367=(
LENGTH_UNIT()
NAMED_UNIT(*)
SI_UNIT(.CENTI.,.METRE.)
);
#73369=(
NAMED_UNIT(*)
PLANE_ANGLE_UNIT()
SI_UNIT($,.RADIAN.)
);
#73370=(
NAMED_UNIT(*)
SI_UNIT($,.STERADIAN.)
SOLID_ANGLE_UNIT()
);
#73400=SHAPE_DEFINITION_REPRESENTATION(#73468,#73636);
#73468=PRODUCT_DEFINITION_SHAPE('',$,#73700);
#73636=SHAPE_REPRESENTATION('',(#17602),#73332);
#73670=PRODUCT_DEFINITION_CONTEXT('part definition',#73861,'design');
#73700=PRODUCT_DEFINITION('Cage (1)','Cage (1)',#73763,#73670);
#73763=PRODUCT_DEFINITION_FORMATION('',$,#73892);
#73861=APPLICATION_CONTEXT(
'Core Data for Automotive Mechanical Design Process');
#73862=PRODUCT_CONTEXT('part definition',#73861,'mechanical');
#73892=PRODUCT('Cage (1)','Cage (1)','Cage (1)',(#73862));
#73982=COLOUR_RGB('Grey',0.48,0.52,0.57);
#73983=FILL_AREA_STYLE_COLOUR('',#73982);
#73984=FILL_AREA_STYLE('',(#73983));
#73985=SURFACE_STYLE_FILL_AREA(#73984);
#73986=SURFACE_SIDE_STYLE('',(#73985));
#73987=SURFACE_STYLE_USAGE(.BOTH.,#73986);
#73988=PRESENTATION_STYLE_ASSIGNMENT((#73987));
ENDSEC;
END-ISO-10303-21;
